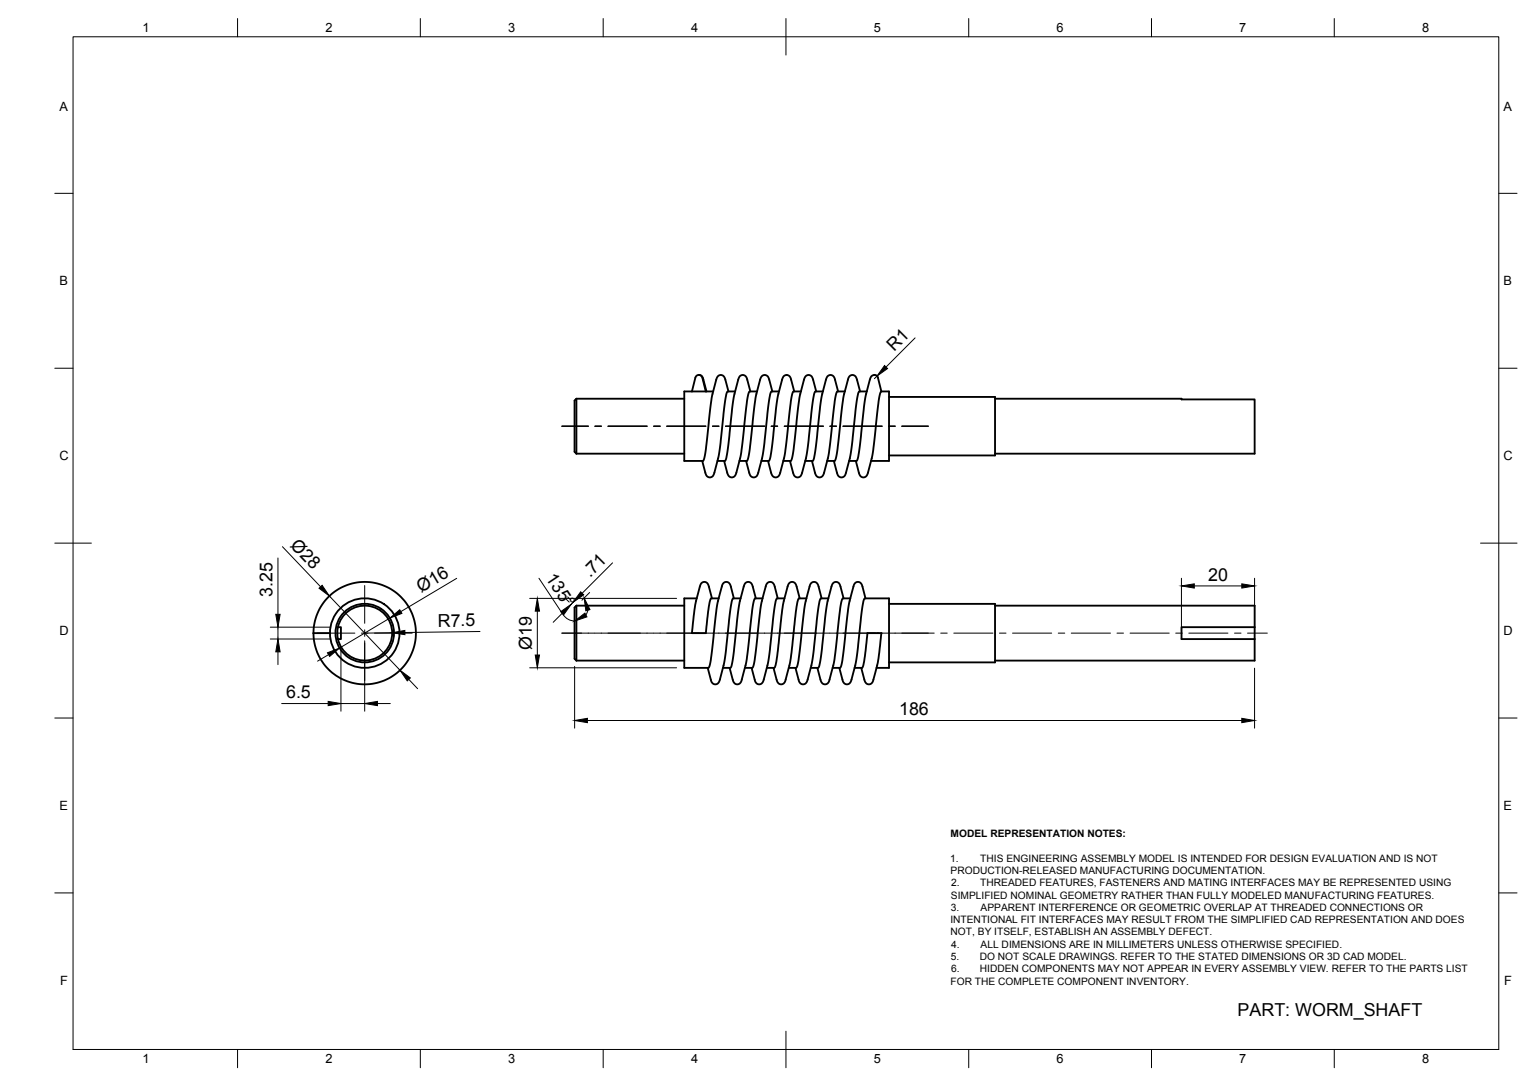
ISO-10303-21;
HEADER;
/* Generated by software containing ST-Developer
 * from STEP Tools, Inc. (www.steptools.com) 
 */

FILE_DESCRIPTION(
/* description */ ('STEP AP214'),
/* implementation_level */ '2;1');

FILE_NAME(
/* name */ 'Worm_Shaft.step',
/* time_stamp */ '2026-10-05T13:15:56-07:00',
/* author */ (''),
/* organization */ (''),
/* preprocessor_version */ 'ST-DEVELOPER v20.2',
/* originating_system */ 'Autodesk Translation Framework v15.15.0.0',
/* authorisation */ '');

FILE_SCHEMA (('AUTOMOTIVE_DESIGN { 1 0 10303 214 3 1 1 }'));
ENDSEC;

DATA;
#10=MECHANICAL_DESIGN_GEOMETRIC_PRESENTATION_REPRESENTATION('',(#1346),#37881);
#228=(
BOUNDED_CURVE()
B_SPLINE_CURVE(2,(#15162,#15163,#15164,#15165,#15166,#15167,#15168,#15169,
#15170,#15171,#15172,#15173,#15174,#15175,#15176,#15177,#15178,#15179,#15180,
#15181,#15182,#15183,#15184,#15185,#15186,#15187,#15188,#15189,#15190,#15191,
#15192,#15193,#15194,#15195,#15196,#15197,#15198,#15199,#15200,#15201,#15202,
#15203,#15204,#15205,#15206,#15207,#15208,#15209,#15210,#15211,#15212,#15213,
#15214,#15215,#15216,#15217,#15218,#15219,#15220,#15221,#15222,#15223,#15224,
#15225,#15226,#15227,#15228,#15229,#15230,#15231,#15232,#15233,#15234,#15235,
#15236,#15237,#15238,#15239,#15240,#15241,#15242,#15243,#15244,#15245,#15246,
#15247,#15248,#15249,#15250,#15251,#15252,#15253,#15254,#15255,#15256,#15257,
#15258,#15259,#15260,#15261,#15262,#15263,#15264,#15265,#15266,#15267,#15268,
#15269,#15270,#15271,#15272,#15273,#15274),.UNSPECIFIED.,.F.,.F.)
B_SPLINE_CURVE_WITH_KNOTS((3,2,2,2,2,2,2,2,2,2,2,2,2,2,2,2,2,2,2,2,2,2,
2,2,2,2,2,2,2,2,2,2,2,2,2,2,2,2,2,2,2,2,2,2,2,2,2,2,2,2,2,2,2,2,2,2,3),
(0.,0.0178571428571429,0.0357142857142857,0.0535714285714286,0.0714285714285714,
0.0892857142857143,0.107142857142857,0.125,0.142857142857143,0.160714285714286,
0.178571428571429,0.196428571428571,0.214285714285714,0.232142857142857,
0.25,0.267857142857143,0.285714285714286,0.303571428571429,0.321428571428571,
0.339285714285714,0.357142857142857,0.375,0.392857142857143,0.410714285714286,
0.428571428571429,0.446428571428571,0.464285714285714,0.482142857142857,
0.5,0.517857142857143,0.535714285714286,0.553571428571429,0.571428571428571,
0.589285714285714,0.607142857142857,0.625,0.642857142857143,0.660714285714286,
0.678571428571429,0.696428571428571,0.714285714285714,0.732142857142857,
0.75,0.767857142857143,0.785714285714286,0.803571428571429,0.821428571428571,
0.839285714285714,0.857142857142857,0.875,0.892857142857143,0.910714285714286,
0.928571428571429,0.946428571428571,0.964285714285714,0.982142857142857,
1.),.UNSPECIFIED.)
CURVE()
GEOMETRIC_REPRESENTATION_ITEM()
RATIONAL_B_SPLINE_CURVE((1.,0.974927912181824,1.,0.974927912181824,1.,0.974927912181824,
1.,0.974927912181824,1.,0.974927912181824,1.,0.974927912181824,1.,0.974927912181824,
1.,0.974927912181824,1.,0.974927912181824,1.,0.974927912181824,1.,0.974927912181824,
1.,0.974927912181824,1.,0.974927912181824,1.,0.974927912181824,1.,0.974927912181824,
1.,0.974927912181824,1.,0.974927912181824,1.,0.974927912181824,1.,0.974927912181824,
1.,0.974927912181824,1.,0.974927912181824,1.,0.974927912181824,1.,0.974927912181824,
1.,0.974927912181824,1.,0.974927912181824,1.,0.974927912181824,1.,0.974927912181824,
1.,0.974927912181824,1.,0.974927912181824,1.,0.974927912181824,1.,0.974927912181824,
1.,0.974927912181824,1.,0.974927912181824,1.,0.974927912181824,1.,0.974927912181824,
1.,0.974927912181824,1.,0.974927912181824,1.,0.974927912181824,1.,0.974927912181824,
1.,0.974927912181824,1.,0.974927912181824,1.,0.974927912181824,1.,0.974927912181824,
1.,0.974927912181824,1.,0.974927912181824,1.,0.974927912181824,1.,0.974927912181824,
1.,0.974927912181824,1.,0.974927912181824,1.,0.974927912181824,1.,0.974927912181824,
1.,0.974927912181824,1.,0.974927912181824,1.,0.974927912181824,1.,0.974927912181824,
1.,0.974927912181824,1.))
REPRESENTATION_ITEM('')
);
#229=(
BOUNDED_CURVE()
B_SPLINE_CURVE(2,(#15729,#15730,#15731,#15732,#15733,#15734,#15735,#15736,
#15737,#15738,#15739,#15740,#15741,#15742,#15743,#15744,#15745,#15746,#15747,
#15748,#15749,#15750,#15751,#15752,#15753,#15754,#15755,#15756,#15757,#15758,
#15759,#15760,#15761,#15762,#15763,#15764,#15765,#15766,#15767,#15768,#15769,
#15770,#15771,#15772,#15773,#15774,#15775,#15776,#15777,#15778,#15779,#15780,
#15781,#15782,#15783,#15784,#15785,#15786,#15787,#15788,#15789,#15790,#15791,
#15792,#15793,#15794,#15795,#15796,#15797,#15798,#15799,#15800,#15801,#15802,
#15803,#15804,#15805,#15806,#15807,#15808,#15809,#15810,#15811,#15812,#15813,
#15814,#15815,#15816,#15817,#15818,#15819,#15820,#15821,#15822,#15823,#15824,
#15825,#15826,#15827,#15828,#15829,#15830,#15831,#15832,#15833,#15834,#15835,
#15836,#15837,#15838,#15839,#15840,#15841),.UNSPECIFIED.,.F.,.F.)
B_SPLINE_CURVE_WITH_KNOTS((3,2,2,2,2,2,2,2,2,2,2,2,2,2,2,2,2,2,2,2,2,2,
2,2,2,2,2,2,2,2,2,2,2,2,2,2,2,2,2,2,2,2,2,2,2,2,2,2,2,2,2,2,2,2,2,2,3),
(0.,0.0178571428571429,0.0357142857142857,0.0535714285714286,0.0714285714285714,
0.0892857142857143,0.107142857142857,0.125,0.142857142857143,0.160714285714286,
0.178571428571429,0.196428571428571,0.214285714285714,0.232142857142857,
0.25,0.267857142857143,0.285714285714286,0.303571428571429,0.321428571428571,
0.339285714285714,0.357142857142857,0.375,0.392857142857143,0.410714285714286,
0.428571428571429,0.446428571428571,0.464285714285714,0.482142857142857,
0.5,0.517857142857143,0.535714285714286,0.553571428571429,0.571428571428571,
0.589285714285714,0.607142857142857,0.625,0.642857142857143,0.660714285714286,
0.678571428571429,0.696428571428571,0.714285714285714,0.732142857142857,
0.75,0.767857142857143,0.785714285714286,0.803571428571429,0.821428571428571,
0.839285714285714,0.857142857142857,0.875,0.892857142857143,0.910714285714286,
0.928571428571429,0.946428571428571,0.964285714285714,0.982142857142857,
1.),.UNSPECIFIED.)
CURVE()
GEOMETRIC_REPRESENTATION_ITEM()
RATIONAL_B_SPLINE_CURVE((1.,0.974927912181824,1.,0.974927912181824,1.,0.974927912181824,
1.,0.974927912181824,1.,0.974927912181824,1.,0.974927912181824,1.,0.974927912181824,
1.,0.974927912181824,1.,0.974927912181824,1.,0.974927912181824,1.,0.974927912181824,
1.,0.974927912181824,1.,0.974927912181824,1.,0.974927912181824,1.,0.974927912181824,
1.,0.974927912181824,1.,0.974927912181824,1.,0.974927912181824,1.,0.974927912181824,
1.,0.974927912181824,1.,0.974927912181824,1.,0.974927912181824,1.,0.974927912181824,
1.,0.974927912181824,1.,0.974927912181824,1.,0.974927912181824,1.,0.974927912181824,
1.,0.974927912181824,1.,0.974927912181824,1.,0.974927912181824,1.,0.974927912181824,
1.,0.974927912181824,1.,0.974927912181824,1.,0.974927912181824,1.,0.974927912181824,
1.,0.974927912181824,1.,0.974927912181824,1.,0.974927912181824,1.,0.974927912181824,
1.,0.974927912181824,1.,0.974927912181824,1.,0.974927912181824,1.,0.974927912181824,
1.,0.974927912181824,1.,0.974927912181824,1.,0.974927912181824,1.,0.974927912181824,
1.,0.974927912181824,1.,0.974927912181824,1.,0.974927912181824,1.,0.974927912181824,
1.,0.974927912181824,1.,0.974927912181824,1.,0.974927912181824,1.,0.974927912181824,
1.,0.974927912181824,1.))
REPRESENTATION_ITEM('')
);
#230=(
BOUNDED_CURVE()
B_SPLINE_CURVE(2,(#16301,#16302,#16303,#16304,#16305,#16306,#16307,#16308,
#16309,#16310,#16311,#16312,#16313,#16314,#16315,#16316,#16317,#16318,#16319,
#16320,#16321,#16322,#16323,#16324,#16325,#16326,#16327,#16328,#16329,#16330,
#16331,#16332,#16333,#16334,#16335,#16336,#16337,#16338,#16339,#16340,#16341,
#16342,#16343,#16344,#16345,#16346,#16347,#16348,#16349,#16350,#16351,#16352,
#16353,#16354,#16355,#16356,#16357,#16358,#16359,#16360,#16361,#16362,#16363,
#16364,#16365,#16366,#16367,#16368,#16369,#16370,#16371,#16372,#16373,#16374,
#16375,#16376,#16377,#16378,#16379,#16380,#16381,#16382,#16383,#16384,#16385,
#16386,#16387,#16388,#16389,#16390,#16391,#16392,#16393,#16394,#16395,#16396,
#16397,#16398,#16399,#16400,#16401,#16402,#16403,#16404,#16405,#16406,#16407,
#16408,#16409,#16410,#16411,#16412,#16413),.UNSPECIFIED.,.F.,.F.)
B_SPLINE_CURVE_WITH_KNOTS((3,2,2,2,2,2,2,2,2,2,2,2,2,2,2,2,2,2,2,2,2,2,
2,2,2,2,2,2,2,2,2,2,2,2,2,2,2,2,2,2,2,2,2,2,2,2,2,2,2,2,2,2,2,2,2,2,3),
(0.,0.0178571428571429,0.0357142857142857,0.0535714285714286,0.0714285714285714,
0.0892857142857143,0.107142857142857,0.125,0.142857142857143,0.160714285714286,
0.178571428571429,0.196428571428571,0.214285714285714,0.232142857142857,
0.25,0.267857142857143,0.285714285714286,0.303571428571429,0.321428571428571,
0.339285714285714,0.357142857142857,0.375,0.392857142857143,0.410714285714286,
0.428571428571429,0.446428571428571,0.464285714285714,0.482142857142857,
0.5,0.517857142857143,0.535714285714286,0.553571428571429,0.571428571428571,
0.589285714285714,0.607142857142857,0.625,0.642857142857143,0.660714285714286,
0.678571428571429,0.696428571428571,0.714285714285714,0.732142857142857,
0.75,0.767857142857143,0.785714285714286,0.803571428571429,0.821428571428571,
0.839285714285714,0.857142857142857,0.875,0.892857142857143,0.910714285714286,
0.928571428571429,0.946428571428571,0.964285714285714,0.982142857142857,
1.),.UNSPECIFIED.)
CURVE()
GEOMETRIC_REPRESENTATION_ITEM()
RATIONAL_B_SPLINE_CURVE((1.,0.974927912181824,1.,0.974927912181824,1.,0.974927912181824,
1.,0.974927912181824,1.,0.974927912181824,1.,0.974927912181824,1.,0.974927912181824,
1.,0.974927912181824,1.,0.974927912181824,1.,0.974927912181824,1.,0.974927912181824,
1.,0.974927912181824,1.,0.974927912181824,1.,0.974927912181824,1.,0.974927912181824,
1.,0.974927912181824,1.,0.974927912181824,1.,0.974927912181824,1.,0.974927912181824,
1.,0.974927912181824,1.,0.974927912181824,1.,0.974927912181824,1.,0.974927912181824,
1.,0.974927912181824,1.,0.974927912181824,1.,0.974927912181824,1.,0.974927912181824,
1.,0.974927912181824,1.,0.974927912181824,1.,0.974927912181824,1.,0.974927912181824,
1.,0.974927912181824,1.,0.974927912181824,1.,0.974927912181824,1.,0.974927912181824,
1.,0.974927912181824,1.,0.974927912181824,1.,0.974927912181824,1.,0.974927912181824,
1.,0.974927912181824,1.,0.974927912181824,1.,0.974927912181824,1.,0.974927912181824,
1.,0.974927912181824,1.,0.974927912181824,1.,0.974927912181824,1.,0.974927912181824,
1.,0.974927912181824,1.,0.974927912181824,1.,0.974927912181824,1.,0.974927912181824,
1.,0.974927912181824,1.,0.974927912181824,1.,0.974927912181824,1.,0.974927912181824,
1.,0.974927912181824,1.))
REPRESENTATION_ITEM('')
);
#231=(
BOUNDED_CURVE()
B_SPLINE_CURVE(2,(#16866,#16867,#16868,#16869,#16870,#16871,#16872,#16873,
#16874,#16875,#16876,#16877,#16878,#16879,#16880,#16881,#16882,#16883,#16884,
#16885,#16886,#16887,#16888,#16889,#16890,#16891,#16892,#16893,#16894,#16895,
#16896,#16897,#16898,#16899,#16900,#16901,#16902,#16903,#16904,#16905,#16906,
#16907,#16908,#16909,#16910,#16911,#16912,#16913,#16914,#16915,#16916,#16917,
#16918,#16919,#16920,#16921,#16922,#16923,#16924,#16925,#16926,#16927,#16928,
#16929,#16930,#16931,#16932,#16933,#16934,#16935,#16936,#16937,#16938,#16939,
#16940,#16941,#16942,#16943,#16944,#16945,#16946,#16947,#16948,#16949,#16950,
#16951,#16952,#16953,#16954,#16955,#16956,#16957,#16958,#16959,#16960,#16961,
#16962,#16963,#16964,#16965,#16966,#16967,#16968,#16969,#16970,#16971,#16972,
#16973,#16974,#16975,#16976,#16977,#16978),.UNSPECIFIED.,.F.,.F.)
B_SPLINE_CURVE_WITH_KNOTS((3,2,2,2,2,2,2,2,2,2,2,2,2,2,2,2,2,2,2,2,2,2,
2,2,2,2,2,2,2,2,2,2,2,2,2,2,2,2,2,2,2,2,2,2,2,2,2,2,2,2,2,2,2,2,2,2,3),
(0.,0.0178571428571429,0.0357142857142857,0.0535714285714286,0.0714285714285714,
0.0892857142857143,0.107142857142857,0.125,0.142857142857143,0.160714285714286,
0.178571428571429,0.196428571428571,0.214285714285714,0.232142857142857,
0.25,0.267857142857143,0.285714285714286,0.303571428571429,0.321428571428571,
0.339285714285714,0.357142857142857,0.375,0.392857142857143,0.410714285714286,
0.428571428571429,0.446428571428571,0.464285714285714,0.482142857142857,
0.5,0.517857142857143,0.535714285714286,0.553571428571429,0.571428571428571,
0.589285714285714,0.607142857142857,0.625,0.642857142857143,0.660714285714286,
0.678571428571429,0.696428571428571,0.714285714285714,0.732142857142857,
0.75,0.767857142857143,0.785714285714286,0.803571428571429,0.821428571428571,
0.839285714285714,0.857142857142857,0.875,0.892857142857143,0.910714285714286,
0.928571428571429,0.946428571428571,0.964285714285714,0.982142857142857,
1.),.UNSPECIFIED.)
CURVE()
GEOMETRIC_REPRESENTATION_ITEM()
RATIONAL_B_SPLINE_CURVE((1.,0.974927912181824,1.,0.974927912181824,1.,0.974927912181824,
1.,0.974927912181824,1.,0.974927912181824,1.,0.974927912181824,1.,0.974927912181824,
1.,0.974927912181824,1.,0.974927912181824,1.,0.974927912181824,1.,0.974927912181824,
1.,0.974927912181824,1.,0.974927912181824,1.,0.974927912181824,1.,0.974927912181824,
1.,0.974927912181824,1.,0.974927912181824,1.,0.974927912181824,1.,0.974927912181824,
1.,0.974927912181824,1.,0.974927912181824,1.,0.974927912181824,1.,0.974927912181824,
1.,0.974927912181824,1.,0.974927912181824,1.,0.974927912181824,1.,0.974927912181824,
1.,0.974927912181824,1.,0.974927912181824,1.,0.974927912181824,1.,0.974927912181824,
1.,0.974927912181824,1.,0.974927912181824,1.,0.974927912181824,1.,0.974927912181824,
1.,0.974927912181824,1.,0.974927912181824,1.,0.974927912181824,1.,0.974927912181824,
1.,0.974927912181824,1.,0.974927912181824,1.,0.974927912181824,1.,0.974927912181824,
1.,0.974927912181824,1.,0.974927912181824,1.,0.974927912181824,1.,0.974927912181824,
1.,0.974927912181824,1.,0.974927912181824,1.,0.974927912181824,1.,0.974927912181824,
1.,0.974927912181824,1.,0.974927912181824,1.,0.974927912181824,1.,0.974927912181824,
1.,0.974927912181824,1.))
REPRESENTATION_ITEM('')
);
#322=(
BOUNDED_SURFACE()
B_SPLINE_SURFACE(1,2,((#14934,#14935,#14936,#14937,#14938,#14939,#14940,
#14941,#14942,#14943,#14944,#14945,#14946,#14947,#14948,#14949,#14950,#14951,
#14952,#14953,#14954,#14955,#14956,#14957,#14958,#14959,#14960,#14961,#14962,
#14963,#14964,#14965,#14966,#14967,#14968,#14969,#14970,#14971,#14972,#14973,
#14974,#14975,#14976,#14977,#14978,#14979,#14980,#14981,#14982,#14983,#14984,
#14985,#14986,#14987,#14988,#14989,#14990,#14991,#14992,#14993,#14994,#14995,
#14996,#14997,#14998,#14999,#15000,#15001,#15002,#15003,#15004,#15005,#15006,
#15007,#15008,#15009,#15010,#15011,#15012,#15013,#15014,#15015,#15016,#15017,
#15018,#15019,#15020,#15021,#15022,#15023,#15024,#15025,#15026,#15027,#15028,
#15029,#15030,#15031,#15032,#15033,#15034,#15035,#15036,#15037,#15038,#15039,
#15040,#15041,#15042,#15043,#15044,#15045,#15046),(#15047,#15048,#15049,
#15050,#15051,#15052,#15053,#15054,#15055,#15056,#15057,#15058,#15059,#15060,
#15061,#15062,#15063,#15064,#15065,#15066,#15067,#15068,#15069,#15070,#15071,
#15072,#15073,#15074,#15075,#15076,#15077,#15078,#15079,#15080,#15081,#15082,
#15083,#15084,#15085,#15086,#15087,#15088,#15089,#15090,#15091,#15092,#15093,
#15094,#15095,#15096,#15097,#15098,#15099,#15100,#15101,#15102,#15103,#15104,
#15105,#15106,#15107,#15108,#15109,#15110,#15111,#15112,#15113,#15114,#15115,
#15116,#15117,#15118,#15119,#15120,#15121,#15122,#15123,#15124,#15125,#15126,
#15127,#15128,#15129,#15130,#15131,#15132,#15133,#15134,#15135,#15136,#15137,
#15138,#15139,#15140,#15141,#15142,#15143,#15144,#15145,#15146,#15147,#15148,
#15149,#15150,#15151,#15152,#15153,#15154,#15155,#15156,#15157,#15158,#15159)),
 .UNSPECIFIED.,.F.,.F.,.F.)
B_SPLINE_SURFACE_WITH_KNOTS((2,2),(3,2,2,2,2,2,2,2,2,2,2,2,2,2,2,2,2,2,
2,2,2,2,2,2,2,2,2,2,2,2,2,2,2,2,2,2,2,2,2,2,2,2,2,2,2,2,2,2,2,2,2,2,2,2,
2,2,3),(0.,1.),(0.,0.0178571428571429,0.0357142857142857,0.0535714285714286,
0.0714285714285714,0.0892857142857143,0.107142857142857,0.125,0.142857142857143,
0.160714285714286,0.178571428571429,0.196428571428571,0.214285714285714,
0.232142857142857,0.25,0.267857142857143,0.285714285714286,0.303571428571429,
0.321428571428571,0.339285714285714,0.357142857142857,0.375,0.392857142857143,
0.410714285714286,0.428571428571429,0.446428571428571,0.464285714285714,
0.482142857142857,0.5,0.517857142857143,0.535714285714286,0.553571428571429,
0.571428571428571,0.589285714285714,0.607142857142857,0.625,0.642857142857143,
0.660714285714286,0.678571428571429,0.696428571428571,0.714285714285714,
0.732142857142857,0.75,0.767857142857143,0.785714285714286,0.803571428571429,
0.821428571428571,0.839285714285714,0.857142857142857,0.875,0.892857142857143,
0.910714285714286,0.928571428571429,0.946428571428571,0.964285714285714,
0.982142857142857,1.),.UNSPECIFIED.)
GEOMETRIC_REPRESENTATION_ITEM()
RATIONAL_B_SPLINE_SURFACE(((1.,0.974927912181824,1.,0.974927912181824,1.,
0.974927912181824,1.,0.974927912181824,1.,0.974927912181824,1.,0.974927912181824,
1.,0.974927912181824,1.,0.974927912181824,1.,0.974927912181824,1.,0.974927912181824,
1.,0.974927912181824,1.,0.974927912181824,1.,0.974927912181824,1.,0.974927912181824,
1.,0.974927912181824,1.,0.974927912181824,1.,0.974927912181824,1.,0.974927912181824,
1.,0.974927912181824,1.,0.974927912181824,1.,0.974927912181824,1.,0.974927912181824,
1.,0.974927912181824,1.,0.974927912181824,1.,0.974927912181824,1.,0.974927912181824,
1.,0.974927912181824,1.,0.974927912181824,1.,0.974927912181824,1.,0.974927912181824,
1.,0.974927912181824,1.,0.974927912181824,1.,0.974927912181824,1.,0.974927912181824,
1.,0.974927912181824,1.,0.974927912181824,1.,0.974927912181824,1.,0.974927912181824,
1.,0.974927912181824,1.,0.974927912181824,1.,0.974927912181824,1.,0.974927912181824,
1.,0.974927912181824,1.,0.974927912181824,1.,0.974927912181824,1.,0.974927912181824,
1.,0.974927912181824,1.,0.974927912181824,1.,0.974927912181824,1.,0.974927912181824,
1.,0.974927912181824,1.,0.974927912181824,1.,0.974927912181824,1.,0.974927912181824,
1.,0.974927912181824,1.,0.974927912181824,1.),(1.,0.974927912181824,1.,
0.974927912181824,1.,0.974927912181824,1.,0.974927912181824,1.,0.974927912181824,
1.,0.974927912181824,1.,0.974927912181824,1.,0.974927912181824,1.,0.974927912181824,
1.,0.974927912181824,1.,0.974927912181824,1.,0.974927912181824,1.,0.974927912181824,
1.,0.974927912181824,1.,0.974927912181824,1.,0.974927912181824,1.,0.974927912181824,
1.,0.974927912181824,1.,0.974927912181824,1.,0.974927912181824,1.,0.974927912181824,
1.,0.974927912181824,1.,0.974927912181824,1.,0.974927912181824,1.,0.974927912181824,
1.,0.974927912181824,1.,0.974927912181824,1.,0.974927912181824,1.,0.974927912181824,
1.,0.974927912181824,1.,0.974927912181824,1.,0.974927912181824,1.,0.974927912181824,
1.,0.974927912181824,1.,0.974927912181824,1.,0.974927912181824,1.,0.974927912181824,
1.,0.974927912181824,1.,0.974927912181824,1.,0.974927912181824,1.,0.974927912181824,
1.,0.974927912181824,1.,0.974927912181824,1.,0.974927912181824,1.,0.974927912181824,
1.,0.974927912181824,1.,0.974927912181824,1.,0.974927912181824,1.,0.974927912181824,
1.,0.974927912181824,1.,0.974927912181824,1.,0.974927912181824,1.,0.974927912181824,
1.,0.974927912181824,1.,0.974927912181824,1.,0.974927912181824,1.)))
REPRESENTATION_ITEM('')
SURFACE()
);
#323=(
BOUNDED_SURFACE()
B_SPLINE_SURFACE(3,2,((#15275,#15276,#15277,#15278,#15279,#15280,#15281,
#15282,#15283,#15284,#15285,#15286,#15287,#15288,#15289,#15290,#15291,#15292,
#15293,#15294,#15295,#15296,#15297,#15298,#15299,#15300,#15301,#15302,#15303,
#15304,#15305,#15306,#15307,#15308,#15309,#15310,#15311,#15312,#15313,#15314,
#15315,#15316,#15317,#15318,#15319,#15320,#15321,#15322,#15323,#15324,#15325,
#15326,#15327,#15328,#15329,#15330,#15331,#15332,#15333,#15334,#15335,#15336,
#15337,#15338,#15339,#15340,#15341,#15342,#15343,#15344,#15345,#15346,#15347,
#15348,#15349,#15350,#15351,#15352,#15353,#15354,#15355,#15356,#15357,#15358,
#15359,#15360,#15361,#15362,#15363,#15364,#15365,#15366,#15367,#15368,#15369,
#15370,#15371,#15372,#15373,#15374,#15375,#15376,#15377,#15378,#15379,#15380,
#15381,#15382,#15383,#15384,#15385,#15386,#15387),(#15388,#15389,#15390,
#15391,#15392,#15393,#15394,#15395,#15396,#15397,#15398,#15399,#15400,#15401,
#15402,#15403,#15404,#15405,#15406,#15407,#15408,#15409,#15410,#15411,#15412,
#15413,#15414,#15415,#15416,#15417,#15418,#15419,#15420,#15421,#15422,#15423,
#15424,#15425,#15426,#15427,#15428,#15429,#15430,#15431,#15432,#15433,#15434,
#15435,#15436,#15437,#15438,#15439,#15440,#15441,#15442,#15443,#15444,#15445,
#15446,#15447,#15448,#15449,#15450,#15451,#15452,#15453,#15454,#15455,#15456,
#15457,#15458,#15459,#15460,#15461,#15462,#15463,#15464,#15465,#15466,#15467,
#15468,#15469,#15470,#15471,#15472,#15473,#15474,#15475,#15476,#15477,#15478,
#15479,#15480,#15481,#15482,#15483,#15484,#15485,#15486,#15487,#15488,#15489,
#15490,#15491,#15492,#15493,#15494,#15495,#15496,#15497,#15498,#15499,#15500),
(#15501,#15502,#15503,#15504,#15505,#15506,#15507,#15508,#15509,#15510,
#15511,#15512,#15513,#15514,#15515,#15516,#15517,#15518,#15519,#15520,#15521,
#15522,#15523,#15524,#15525,#15526,#15527,#15528,#15529,#15530,#15531,#15532,
#15533,#15534,#15535,#15536,#15537,#15538,#15539,#15540,#15541,#15542,#15543,
#15544,#15545,#15546,#15547,#15548,#15549,#15550,#15551,#15552,#15553,#15554,
#15555,#15556,#15557,#15558,#15559,#15560,#15561,#15562,#15563,#15564,#15565,
#15566,#15567,#15568,#15569,#15570,#15571,#15572,#15573,#15574,#15575,#15576,
#15577,#15578,#15579,#15580,#15581,#15582,#15583,#15584,#15585,#15586,#15587,
#15588,#15589,#15590,#15591,#15592,#15593,#15594,#15595,#15596,#15597,#15598,
#15599,#15600,#15601,#15602,#15603,#15604,#15605,#15606,#15607,#15608,#15609,
#15610,#15611,#15612,#15613),(#15614,#15615,#15616,#15617,#15618,#15619,
#15620,#15621,#15622,#15623,#15624,#15625,#15626,#15627,#15628,#15629,#15630,
#15631,#15632,#15633,#15634,#15635,#15636,#15637,#15638,#15639,#15640,#15641,
#15642,#15643,#15644,#15645,#15646,#15647,#15648,#15649,#15650,#15651,#15652,
#15653,#15654,#15655,#15656,#15657,#15658,#15659,#15660,#15661,#15662,#15663,
#15664,#15665,#15666,#15667,#15668,#15669,#15670,#15671,#15672,#15673,#15674,
#15675,#15676,#15677,#15678,#15679,#15680,#15681,#15682,#15683,#15684,#15685,
#15686,#15687,#15688,#15689,#15690,#15691,#15692,#15693,#15694,#15695,#15696,
#15697,#15698,#15699,#15700,#15701,#15702,#15703,#15704,#15705,#15706,#15707,
#15708,#15709,#15710,#15711,#15712,#15713,#15714,#15715,#15716,#15717,#15718,
#15719,#15720,#15721,#15722,#15723,#15724,#15725,#15726)),.UNSPECIFIED.,
 .F.,.F.,.F.)
B_SPLINE_SURFACE_WITH_KNOTS((4,4),(3,2,2,2,2,2,2,2,2,2,2,2,2,2,2,2,2,2,
2,2,2,2,2,2,2,2,2,2,2,2,2,2,2,2,2,2,2,2,2,2,2,2,2,2,2,2,2,2,2,2,2,2,2,2,
2,2,3),(0.,1.),(0.,0.0178571428571429,0.0357142857142857,0.0535714285714286,
0.0714285714285714,0.0892857142857143,0.107142857142857,0.125,0.142857142857143,
0.160714285714286,0.178571428571429,0.196428571428571,0.214285714285714,
0.232142857142857,0.25,0.267857142857143,0.285714285714286,0.303571428571429,
0.321428571428571,0.339285714285714,0.357142857142857,0.375,0.392857142857143,
0.410714285714286,0.428571428571429,0.446428571428571,0.464285714285714,
0.482142857142857,0.5,0.517857142857143,0.535714285714286,0.553571428571429,
0.571428571428571,0.589285714285714,0.607142857142857,0.625,0.642857142857143,
0.660714285714286,0.678571428571429,0.696428571428571,0.714285714285714,
0.732142857142857,0.75,0.767857142857143,0.785714285714286,0.803571428571429,
0.821428571428571,0.839285714285714,0.857142857142857,0.875,0.892857142857143,
0.910714285714286,0.928571428571429,0.946428571428571,0.964285714285714,
0.982142857142857,1.),.UNSPECIFIED.)
GEOMETRIC_REPRESENTATION_ITEM()
RATIONAL_B_SPLINE_SURFACE(((1.,0.974927912181824,1.,0.974927912181824,1.,
0.974927912181824,1.,0.974927912181824,1.,0.974927912181824,1.,0.974927912181824,
1.,0.974927912181824,1.,0.974927912181824,1.,0.974927912181824,1.,0.974927912181824,
1.,0.974927912181824,1.,0.974927912181824,1.,0.974927912181824,1.,0.974927912181824,
1.,0.974927912181824,1.,0.974927912181824,1.,0.974927912181824,1.,0.974927912181824,
1.,0.974927912181824,1.,0.974927912181824,1.,0.974927912181824,1.,0.974927912181824,
1.,0.974927912181824,1.,0.974927912181824,1.,0.974927912181824,1.,0.974927912181824,
1.,0.974927912181824,1.,0.974927912181824,1.,0.974927912181824,1.,0.974927912181824,
1.,0.974927912181824,1.,0.974927912181824,1.,0.974927912181824,1.,0.974927912181824,
1.,0.974927912181824,1.,0.974927912181824,1.,0.974927912181824,1.,0.974927912181824,
1.,0.974927912181824,1.,0.974927912181824,1.,0.974927912181824,1.,0.974927912181824,
1.,0.974927912181824,1.,0.974927912181824,1.,0.974927912181824,1.,0.974927912181824,
1.,0.974927912181824,1.,0.974927912181824,1.,0.974927912181824,1.,0.974927912181824,
1.,0.974927912181824,1.,0.974927912181824,1.,0.974927912181824,1.,0.974927912181824,
1.,0.974927912181824,1.,0.974927912181824,1.),(0.49408353936993,0.481695833481332,
0.49408353936993,0.481695833481332,0.49408353936993,0.481695833481332,0.49408353936993,
0.481695833481332,0.49408353936993,0.481695833481332,0.49408353936993,0.481695833481332,
0.49408353936993,0.481695833481332,0.49408353936993,0.481695833481332,0.49408353936993,
0.481695833481332,0.49408353936993,0.481695833481332,0.49408353936993,0.481695833481332,
0.49408353936993,0.481695833481332,0.49408353936993,0.481695833481332,0.49408353936993,
0.481695833481332,0.49408353936993,0.481695833481332,0.49408353936993,0.481695833481332,
0.49408353936993,0.481695833481332,0.49408353936993,0.481695833481332,0.49408353936993,
0.481695833481332,0.49408353936993,0.481695833481332,0.49408353936993,0.481695833481332,
0.49408353936993,0.481695833481332,0.49408353936993,0.481695833481332,0.49408353936993,
0.481695833481332,0.49408353936993,0.481695833481332,0.49408353936993,0.481695833481332,
0.49408353936993,0.481695833481332,0.49408353936993,0.481695833481332,0.49408353936993,
0.481695833481332,0.49408353936993,0.481695833481332,0.49408353936993,0.481695833481332,
0.49408353936993,0.481695833481332,0.49408353936993,0.481695833481332,0.49408353936993,
0.481695833481332,0.49408353936993,0.481695833481332,0.49408353936993,0.481695833481332,
0.49408353936993,0.481695833481332,0.49408353936993,0.481695833481332,0.49408353936993,
0.481695833481332,0.49408353936993,0.481695833481332,0.49408353936993,0.481695833481332,
0.49408353936993,0.481695833481332,0.49408353936993,0.481695833481332,0.49408353936993,
0.481695833481332,0.49408353936993,0.481695833481332,0.49408353936993,0.481695833481332,
0.49408353936993,0.481695833481332,0.49408353936993,0.481695833481332,0.49408353936993,
0.481695833481332,0.49408353936993,0.481695833481332,0.49408353936993,0.481695833481332,
0.49408353936993,0.481695833481332,0.49408353936993,0.481695833481332,0.49408353936993,
0.481695833481332,0.49408353936993,0.481695833481332,0.49408353936993,0.481695833481332,
0.49408353936993),(0.49408353936993,0.481695833481332,0.49408353936993,
0.481695833481332,0.49408353936993,0.481695833481332,0.49408353936993,0.481695833481332,
0.49408353936993,0.481695833481332,0.49408353936993,0.481695833481332,0.49408353936993,
0.481695833481332,0.49408353936993,0.481695833481332,0.49408353936993,0.481695833481332,
0.49408353936993,0.481695833481332,0.49408353936993,0.481695833481332,0.49408353936993,
0.481695833481332,0.49408353936993,0.481695833481332,0.49408353936993,0.481695833481332,
0.49408353936993,0.481695833481332,0.49408353936993,0.481695833481332,0.49408353936993,
0.481695833481332,0.49408353936993,0.481695833481332,0.49408353936993,0.481695833481332,
0.49408353936993,0.481695833481332,0.49408353936993,0.481695833481332,0.49408353936993,
0.481695833481332,0.49408353936993,0.481695833481332,0.49408353936993,0.481695833481332,
0.49408353936993,0.481695833481332,0.49408353936993,0.481695833481332,0.49408353936993,
0.481695833481332,0.49408353936993,0.481695833481332,0.49408353936993,0.481695833481332,
0.49408353936993,0.481695833481332,0.49408353936993,0.481695833481332,0.49408353936993,
0.481695833481332,0.49408353936993,0.481695833481332,0.49408353936993,0.481695833481332,
0.49408353936993,0.481695833481332,0.49408353936993,0.481695833481332,0.49408353936993,
0.481695833481332,0.49408353936993,0.481695833481332,0.49408353936993,0.481695833481332,
0.49408353936993,0.481695833481332,0.49408353936993,0.481695833481332,0.49408353936993,
0.481695833481332,0.49408353936993,0.481695833481332,0.49408353936993,0.481695833481332,
0.49408353936993,0.481695833481332,0.49408353936993,0.481695833481332,0.49408353936993,
0.481695833481332,0.49408353936993,0.481695833481332,0.49408353936993,0.481695833481332,
0.49408353936993,0.481695833481332,0.49408353936993,0.481695833481332,0.49408353936993,
0.481695833481332,0.49408353936993,0.481695833481332,0.49408353936993,0.481695833481332,
0.49408353936993,0.481695833481332,0.49408353936993,0.481695833481332,0.49408353936993),
(1.,0.974927912181824,1.,0.974927912181824,1.,0.974927912181824,1.,0.974927912181824,
1.,0.974927912181824,1.,0.974927912181824,1.,0.974927912181824,1.,0.974927912181824,
1.,0.974927912181824,1.,0.974927912181824,1.,0.974927912181824,1.,0.974927912181824,
1.,0.974927912181824,1.,0.974927912181824,1.,0.974927912181824,1.,0.974927912181824,
1.,0.974927912181824,1.,0.974927912181824,1.,0.974927912181824,1.,0.974927912181824,
1.,0.974927912181824,1.,0.974927912181824,1.,0.974927912181824,1.,0.974927912181824,
1.,0.974927912181824,1.,0.974927912181824,1.,0.974927912181824,1.,0.974927912181824,
1.,0.974927912181824,1.,0.974927912181824,1.,0.974927912181824,1.,0.974927912181824,
1.,0.974927912181824,1.,0.974927912181824,1.,0.974927912181824,1.,0.974927912181824,
1.,0.974927912181824,1.,0.974927912181824,1.,0.974927912181824,1.,0.974927912181824,
1.,0.974927912181824,1.,0.974927912181824,1.,0.974927912181824,1.,0.974927912181824,
1.,0.974927912181824,1.,0.974927912181824,1.,0.974927912181824,1.,0.974927912181824,
1.,0.974927912181824,1.,0.974927912181824,1.,0.974927912181824,1.,0.974927912181824,
1.,0.974927912181824,1.,0.974927912181824,1.,0.974927912181824,1.,0.974927912181824,
1.)))
REPRESENTATION_ITEM('')
SURFACE()
);
#324=(
BOUNDED_SURFACE()
B_SPLINE_SURFACE(1,2,((#15842,#15843,#15844,#15845,#15846,#15847,#15848,
#15849,#15850,#15851,#15852,#15853,#15854,#15855,#15856,#15857,#15858,#15859,
#15860,#15861,#15862,#15863,#15864,#15865,#15866,#15867,#15868,#15869,#15870,
#15871,#15872,#15873,#15874,#15875,#15876,#15877,#15878,#15879,#15880,#15881,
#15882,#15883,#15884,#15885,#15886,#15887,#15888,#15889,#15890,#15891,#15892,
#15893,#15894,#15895,#15896,#15897,#15898,#15899,#15900,#15901,#15902,#15903,
#15904,#15905,#15906,#15907,#15908,#15909,#15910,#15911,#15912,#15913,#15914,
#15915,#15916,#15917,#15918,#15919,#15920,#15921,#15922,#15923,#15924,#15925,
#15926,#15927,#15928,#15929,#15930,#15931,#15932,#15933,#15934,#15935,#15936,
#15937,#15938,#15939,#15940,#15941,#15942,#15943,#15944,#15945,#15946,#15947,
#15948,#15949,#15950,#15951,#15952,#15953,#15954),(#15955,#15956,#15957,
#15958,#15959,#15960,#15961,#15962,#15963,#15964,#15965,#15966,#15967,#15968,
#15969,#15970,#15971,#15972,#15973,#15974,#15975,#15976,#15977,#15978,#15979,
#15980,#15981,#15982,#15983,#15984,#15985,#15986,#15987,#15988,#15989,#15990,
#15991,#15992,#15993,#15994,#15995,#15996,#15997,#15998,#15999,#16000,#16001,
#16002,#16003,#16004,#16005,#16006,#16007,#16008,#16009,#16010,#16011,#16012,
#16013,#16014,#16015,#16016,#16017,#16018,#16019,#16020,#16021,#16022,#16023,
#16024,#16025,#16026,#16027,#16028,#16029,#16030,#16031,#16032,#16033,#16034,
#16035,#16036,#16037,#16038,#16039,#16040,#16041,#16042,#16043,#16044,#16045,
#16046,#16047,#16048,#16049,#16050,#16051,#16052,#16053,#16054,#16055,#16056,
#16057,#16058,#16059,#16060,#16061,#16062,#16063,#16064,#16065,#16066,#16067)),
 .UNSPECIFIED.,.F.,.F.,.F.)
B_SPLINE_SURFACE_WITH_KNOTS((2,2),(3,2,2,2,2,2,2,2,2,2,2,2,2,2,2,2,2,2,
2,2,2,2,2,2,2,2,2,2,2,2,2,2,2,2,2,2,2,2,2,2,2,2,2,2,2,2,2,2,2,2,2,2,2,2,
2,2,3),(0.,1.),(0.,0.0178571428571429,0.0357142857142857,0.0535714285714286,
0.0714285714285714,0.0892857142857143,0.107142857142857,0.125,0.142857142857143,
0.160714285714286,0.178571428571429,0.196428571428571,0.214285714285714,
0.232142857142857,0.25,0.267857142857143,0.285714285714286,0.303571428571429,
0.321428571428571,0.339285714285714,0.357142857142857,0.375,0.392857142857143,
0.410714285714286,0.428571428571429,0.446428571428571,0.464285714285714,
0.482142857142857,0.5,0.517857142857143,0.535714285714286,0.553571428571429,
0.571428571428571,0.589285714285714,0.607142857142857,0.625,0.642857142857143,
0.660714285714286,0.678571428571429,0.696428571428571,0.714285714285714,
0.732142857142857,0.75,0.767857142857143,0.785714285714286,0.803571428571429,
0.821428571428571,0.839285714285714,0.857142857142857,0.875,0.892857142857143,
0.910714285714286,0.928571428571429,0.946428571428571,0.964285714285714,
0.982142857142857,1.),.UNSPECIFIED.)
GEOMETRIC_REPRESENTATION_ITEM()
RATIONAL_B_SPLINE_SURFACE(((1.,0.974927912181824,1.,0.974927912181824,1.,
0.974927912181824,1.,0.974927912181824,1.,0.974927912181824,1.,0.974927912181824,
1.,0.974927912181824,1.,0.974927912181824,1.,0.974927912181824,1.,0.974927912181824,
1.,0.974927912181824,1.,0.974927912181824,1.,0.974927912181824,1.,0.974927912181824,
1.,0.974927912181824,1.,0.974927912181824,1.,0.974927912181824,1.,0.974927912181824,
1.,0.974927912181824,1.,0.974927912181824,1.,0.974927912181824,1.,0.974927912181824,
1.,0.974927912181824,1.,0.974927912181824,1.,0.974927912181824,1.,0.974927912181824,
1.,0.974927912181824,1.,0.974927912181824,1.,0.974927912181824,1.,0.974927912181824,
1.,0.974927912181824,1.,0.974927912181824,1.,0.974927912181824,1.,0.974927912181824,
1.,0.974927912181824,1.,0.974927912181824,1.,0.974927912181824,1.,0.974927912181824,
1.,0.974927912181824,1.,0.974927912181824,1.,0.974927912181824,1.,0.974927912181824,
1.,0.974927912181824,1.,0.974927912181824,1.,0.974927912181824,1.,0.974927912181824,
1.,0.974927912181824,1.,0.974927912181824,1.,0.974927912181824,1.,0.974927912181824,
1.,0.974927912181824,1.,0.974927912181824,1.,0.974927912181824,1.,0.974927912181824,
1.,0.974927912181824,1.,0.974927912181824,1.),(1.,0.974927912181824,1.,
0.974927912181824,1.,0.974927912181824,1.,0.974927912181824,1.,0.974927912181824,
1.,0.974927912181824,1.,0.974927912181824,1.,0.974927912181824,1.,0.974927912181824,
1.,0.974927912181824,1.,0.974927912181824,1.,0.974927912181824,1.,0.974927912181824,
1.,0.974927912181824,1.,0.974927912181824,1.,0.974927912181824,1.,0.974927912181824,
1.,0.974927912181824,1.,0.974927912181824,1.,0.974927912181824,1.,0.974927912181824,
1.,0.974927912181824,1.,0.974927912181824,1.,0.974927912181824,1.,0.974927912181824,
1.,0.974927912181824,1.,0.974927912181824,1.,0.974927912181824,1.,0.974927912181824,
1.,0.974927912181824,1.,0.974927912181824,1.,0.974927912181824,1.,0.974927912181824,
1.,0.974927912181824,1.,0.974927912181824,1.,0.974927912181824,1.,0.974927912181824,
1.,0.974927912181824,1.,0.974927912181824,1.,0.974927912181824,1.,0.974927912181824,
1.,0.974927912181824,1.,0.974927912181824,1.,0.974927912181824,1.,0.974927912181824,
1.,0.974927912181824,1.,0.974927912181824,1.,0.974927912181824,1.,0.974927912181824,
1.,0.974927912181824,1.,0.974927912181824,1.,0.974927912181824,1.,0.974927912181824,
1.,0.974927912181824,1.,0.974927912181824,1.,0.974927912181824,1.)))
REPRESENTATION_ITEM('')
SURFACE()
);
#325=(
BOUNDED_SURFACE()
B_SPLINE_SURFACE(1,2,((#16075,#16076,#16077,#16078,#16079,#16080,#16081,
#16082,#16083,#16084,#16085,#16086,#16087,#16088,#16089,#16090,#16091,#16092,
#16093,#16094,#16095,#16096,#16097,#16098,#16099,#16100,#16101,#16102,#16103,
#16104,#16105,#16106,#16107,#16108,#16109,#16110,#16111,#16112,#16113,#16114,
#16115,#16116,#16117,#16118,#16119,#16120,#16121,#16122,#16123,#16124,#16125,
#16126,#16127,#16128,#16129,#16130,#16131,#16132,#16133,#16134,#16135,#16136,
#16137,#16138,#16139,#16140,#16141,#16142,#16143,#16144,#16145,#16146,#16147,
#16148,#16149,#16150,#16151,#16152,#16153,#16154,#16155,#16156,#16157,#16158,
#16159,#16160,#16161,#16162,#16163,#16164,#16165,#16166,#16167,#16168,#16169,
#16170,#16171,#16172,#16173,#16174,#16175,#16176,#16177,#16178,#16179,#16180,
#16181,#16182,#16183,#16184,#16185,#16186,#16187),(#16188,#16189,#16190,
#16191,#16192,#16193,#16194,#16195,#16196,#16197,#16198,#16199,#16200,#16201,
#16202,#16203,#16204,#16205,#16206,#16207,#16208,#16209,#16210,#16211,#16212,
#16213,#16214,#16215,#16216,#16217,#16218,#16219,#16220,#16221,#16222,#16223,
#16224,#16225,#16226,#16227,#16228,#16229,#16230,#16231,#16232,#16233,#16234,
#16235,#16236,#16237,#16238,#16239,#16240,#16241,#16242,#16243,#16244,#16245,
#16246,#16247,#16248,#16249,#16250,#16251,#16252,#16253,#16254,#16255,#16256,
#16257,#16258,#16259,#16260,#16261,#16262,#16263,#16264,#16265,#16266,#16267,
#16268,#16269,#16270,#16271,#16272,#16273,#16274,#16275,#16276,#16277,#16278,
#16279,#16280,#16281,#16282,#16283,#16284,#16285,#16286,#16287,#16288,#16289,
#16290,#16291,#16292,#16293,#16294,#16295,#16296,#16297,#16298,#16299,#16300)),
 .UNSPECIFIED.,.F.,.F.,.F.)
B_SPLINE_SURFACE_WITH_KNOTS((2,2),(3,2,2,2,2,2,2,2,2,2,2,2,2,2,2,2,2,2,
2,2,2,2,2,2,2,2,2,2,2,2,2,2,2,2,2,2,2,2,2,2,2,2,2,2,2,2,2,2,2,2,2,2,2,2,
2,2,3),(0.,1.),(0.,0.0178571428571429,0.0357142857142857,0.0535714285714286,
0.0714285714285714,0.0892857142857143,0.107142857142857,0.125,0.142857142857143,
0.160714285714286,0.178571428571429,0.196428571428571,0.214285714285714,
0.232142857142857,0.25,0.267857142857143,0.285714285714286,0.303571428571429,
0.321428571428571,0.339285714285714,0.357142857142857,0.375,0.392857142857143,
0.410714285714286,0.428571428571429,0.446428571428571,0.464285714285714,
0.482142857142857,0.5,0.517857142857143,0.535714285714286,0.553571428571429,
0.571428571428571,0.589285714285714,0.607142857142857,0.625,0.642857142857143,
0.660714285714286,0.678571428571429,0.696428571428571,0.714285714285714,
0.732142857142857,0.75,0.767857142857143,0.785714285714286,0.803571428571429,
0.821428571428571,0.839285714285714,0.857142857142857,0.875,0.892857142857143,
0.910714285714286,0.928571428571429,0.946428571428571,0.964285714285714,
0.982142857142857,1.),.UNSPECIFIED.)
GEOMETRIC_REPRESENTATION_ITEM()
RATIONAL_B_SPLINE_SURFACE(((1.,0.974927912181824,1.,0.974927912181824,1.,
0.974927912181824,1.,0.974927912181824,1.,0.974927912181824,1.,0.974927912181824,
1.,0.974927912181824,1.,0.974927912181824,1.,0.974927912181824,1.,0.974927912181824,
1.,0.974927912181824,1.,0.974927912181824,1.,0.974927912181824,1.,0.974927912181824,
1.,0.974927912181824,1.,0.974927912181824,1.,0.974927912181824,1.,0.974927912181824,
1.,0.974927912181824,1.,0.974927912181824,1.,0.974927912181824,1.,0.974927912181824,
1.,0.974927912181824,1.,0.974927912181824,1.,0.974927912181824,1.,0.974927912181824,
1.,0.974927912181824,1.,0.974927912181824,1.,0.974927912181824,1.,0.974927912181824,
1.,0.974927912181824,1.,0.974927912181824,1.,0.974927912181824,1.,0.974927912181824,
1.,0.974927912181824,1.,0.974927912181824,1.,0.974927912181824,1.,0.974927912181824,
1.,0.974927912181824,1.,0.974927912181824,1.,0.974927912181824,1.,0.974927912181824,
1.,0.974927912181824,1.,0.974927912181824,1.,0.974927912181824,1.,0.974927912181824,
1.,0.974927912181824,1.,0.974927912181824,1.,0.974927912181824,1.,0.974927912181824,
1.,0.974927912181824,1.,0.974927912181824,1.,0.974927912181824,1.,0.974927912181824,
1.,0.974927912181824,1.,0.974927912181824,1.),(1.,0.974927912181824,1.,
0.974927912181824,1.,0.974927912181824,1.,0.974927912181824,1.,0.974927912181824,
1.,0.974927912181824,1.,0.974927912181824,1.,0.974927912181824,1.,0.974927912181824,
1.,0.974927912181824,1.,0.974927912181824,1.,0.974927912181824,1.,0.974927912181824,
1.,0.974927912181824,1.,0.974927912181824,1.,0.974927912181824,1.,0.974927912181824,
1.,0.974927912181824,1.,0.974927912181824,1.,0.974927912181824,1.,0.974927912181824,
1.,0.974927912181824,1.,0.974927912181824,1.,0.974927912181824,1.,0.974927912181824,
1.,0.974927912181824,1.,0.974927912181824,1.,0.974927912181824,1.,0.974927912181824,
1.,0.974927912181824,1.,0.974927912181824,1.,0.974927912181824,1.,0.974927912181824,
1.,0.974927912181824,1.,0.974927912181824,1.,0.974927912181824,1.,0.974927912181824,
1.,0.974927912181824,1.,0.974927912181824,1.,0.974927912181824,1.,0.974927912181824,
1.,0.974927912181824,1.,0.974927912181824,1.,0.974927912181824,1.,0.974927912181824,
1.,0.974927912181824,1.,0.974927912181824,1.,0.974927912181824,1.,0.974927912181824,
1.,0.974927912181824,1.,0.974927912181824,1.,0.974927912181824,1.,0.974927912181824,
1.,0.974927912181824,1.,0.974927912181824,1.,0.974927912181824,1.)))
REPRESENTATION_ITEM('')
SURFACE()
);
#326=(
BOUNDED_SURFACE()
B_SPLINE_SURFACE(3,2,((#16414,#16415,#16416,#16417,#16418,#16419,#16420,
#16421,#16422,#16423,#16424,#16425,#16426,#16427,#16428,#16429,#16430,#16431,
#16432,#16433,#16434,#16435,#16436,#16437,#16438,#16439,#16440,#16441,#16442,
#16443,#16444,#16445,#16446,#16447,#16448,#16449,#16450,#16451,#16452,#16453,
#16454,#16455,#16456,#16457,#16458,#16459,#16460,#16461,#16462,#16463,#16464,
#16465,#16466,#16467,#16468,#16469,#16470,#16471,#16472,#16473,#16474,#16475,
#16476,#16477,#16478,#16479,#16480,#16481,#16482,#16483,#16484,#16485,#16486,
#16487,#16488,#16489,#16490,#16491,#16492,#16493,#16494,#16495,#16496,#16497,
#16498,#16499,#16500,#16501,#16502,#16503,#16504,#16505,#16506,#16507,#16508,
#16509,#16510,#16511,#16512,#16513,#16514,#16515,#16516,#16517,#16518,#16519,
#16520,#16521,#16522,#16523,#16524,#16525,#16526),(#16527,#16528,#16529,
#16530,#16531,#16532,#16533,#16534,#16535,#16536,#16537,#16538,#16539,#16540,
#16541,#16542,#16543,#16544,#16545,#16546,#16547,#16548,#16549,#16550,#16551,
#16552,#16553,#16554,#16555,#16556,#16557,#16558,#16559,#16560,#16561,#16562,
#16563,#16564,#16565,#16566,#16567,#16568,#16569,#16570,#16571,#16572,#16573,
#16574,#16575,#16576,#16577,#16578,#16579,#16580,#16581,#16582,#16583,#16584,
#16585,#16586,#16587,#16588,#16589,#16590,#16591,#16592,#16593,#16594,#16595,
#16596,#16597,#16598,#16599,#16600,#16601,#16602,#16603,#16604,#16605,#16606,
#16607,#16608,#16609,#16610,#16611,#16612,#16613,#16614,#16615,#16616,#16617,
#16618,#16619,#16620,#16621,#16622,#16623,#16624,#16625,#16626,#16627,#16628,
#16629,#16630,#16631,#16632,#16633,#16634,#16635,#16636,#16637,#16638,#16639),
(#16640,#16641,#16642,#16643,#16644,#16645,#16646,#16647,#16648,#16649,
#16650,#16651,#16652,#16653,#16654,#16655,#16656,#16657,#16658,#16659,#16660,
#16661,#16662,#16663,#16664,#16665,#16666,#16667,#16668,#16669,#16670,#16671,
#16672,#16673,#16674,#16675,#16676,#16677,#16678,#16679,#16680,#16681,#16682,
#16683,#16684,#16685,#16686,#16687,#16688,#16689,#16690,#16691,#16692,#16693,
#16694,#16695,#16696,#16697,#16698,#16699,#16700,#16701,#16702,#16703,#16704,
#16705,#16706,#16707,#16708,#16709,#16710,#16711,#16712,#16713,#16714,#16715,
#16716,#16717,#16718,#16719,#16720,#16721,#16722,#16723,#16724,#16725,#16726,
#16727,#16728,#16729,#16730,#16731,#16732,#16733,#16734,#16735,#16736,#16737,
#16738,#16739,#16740,#16741,#16742,#16743,#16744,#16745,#16746,#16747,#16748,
#16749,#16750,#16751,#16752),(#16753,#16754,#16755,#16756,#16757,#16758,
#16759,#16760,#16761,#16762,#16763,#16764,#16765,#16766,#16767,#16768,#16769,
#16770,#16771,#16772,#16773,#16774,#16775,#16776,#16777,#16778,#16779,#16780,
#16781,#16782,#16783,#16784,#16785,#16786,#16787,#16788,#16789,#16790,#16791,
#16792,#16793,#16794,#16795,#16796,#16797,#16798,#16799,#16800,#16801,#16802,
#16803,#16804,#16805,#16806,#16807,#16808,#16809,#16810,#16811,#16812,#16813,
#16814,#16815,#16816,#16817,#16818,#16819,#16820,#16821,#16822,#16823,#16824,
#16825,#16826,#16827,#16828,#16829,#16830,#16831,#16832,#16833,#16834,#16835,
#16836,#16837,#16838,#16839,#16840,#16841,#16842,#16843,#16844,#16845,#16846,
#16847,#16848,#16849,#16850,#16851,#16852,#16853,#16854,#16855,#16856,#16857,
#16858,#16859,#16860,#16861,#16862,#16863,#16864,#16865)),.UNSPECIFIED.,
 .F.,.F.,.F.)
B_SPLINE_SURFACE_WITH_KNOTS((4,4),(3,2,2,2,2,2,2,2,2,2,2,2,2,2,2,2,2,2,
2,2,2,2,2,2,2,2,2,2,2,2,2,2,2,2,2,2,2,2,2,2,2,2,2,2,2,2,2,2,2,2,2,2,2,2,
2,2,3),(0.,1.),(0.,0.0178571428571429,0.0357142857142857,0.0535714285714286,
0.0714285714285714,0.0892857142857143,0.107142857142857,0.125,0.142857142857143,
0.160714285714286,0.178571428571429,0.196428571428571,0.214285714285714,
0.232142857142857,0.25,0.267857142857143,0.285714285714286,0.303571428571429,
0.321428571428571,0.339285714285714,0.357142857142857,0.375,0.392857142857143,
0.410714285714286,0.428571428571429,0.446428571428571,0.464285714285714,
0.482142857142857,0.5,0.517857142857143,0.535714285714286,0.553571428571429,
0.571428571428571,0.589285714285714,0.607142857142857,0.625,0.642857142857143,
0.660714285714286,0.678571428571429,0.696428571428571,0.714285714285714,
0.732142857142857,0.75,0.767857142857143,0.785714285714286,0.803571428571429,
0.821428571428571,0.839285714285714,0.857142857142857,0.875,0.892857142857143,
0.910714285714286,0.928571428571429,0.946428571428571,0.964285714285714,
0.982142857142857,1.),.UNSPECIFIED.)
GEOMETRIC_REPRESENTATION_ITEM()
RATIONAL_B_SPLINE_SURFACE(((1.,0.974927912181824,1.,0.974927912181824,1.,
0.974927912181824,1.,0.974927912181824,1.,0.974927912181824,1.,0.974927912181824,
1.,0.974927912181824,1.,0.974927912181824,1.,0.974927912181824,1.,0.974927912181824,
1.,0.974927912181824,1.,0.974927912181824,1.,0.974927912181824,1.,0.974927912181824,
1.,0.974927912181824,1.,0.974927912181824,1.,0.974927912181824,1.,0.974927912181824,
1.,0.974927912181824,1.,0.974927912181824,1.,0.974927912181824,1.,0.974927912181824,
1.,0.974927912181824,1.,0.974927912181824,1.,0.974927912181824,1.,0.974927912181824,
1.,0.974927912181824,1.,0.974927912181824,1.,0.974927912181824,1.,0.974927912181824,
1.,0.974927912181824,1.,0.974927912181824,1.,0.974927912181824,1.,0.974927912181824,
1.,0.974927912181824,1.,0.974927912181824,1.,0.974927912181824,1.,0.974927912181824,
1.,0.974927912181824,1.,0.974927912181824,1.,0.974927912181824,1.,0.974927912181824,
1.,0.974927912181824,1.,0.974927912181824,1.,0.974927912181824,1.,0.974927912181824,
1.,0.974927912181824,1.,0.974927912181824,1.,0.974927912181824,1.,0.974927912181824,
1.,0.974927912181824,1.,0.974927912181824,1.,0.974927912181824,1.,0.974927912181824,
1.,0.974927912181824,1.,0.974927912181824,1.),(0.49408353936993,0.481695833481332,
0.49408353936993,0.481695833481332,0.49408353936993,0.481695833481332,0.49408353936993,
0.481695833481332,0.49408353936993,0.481695833481332,0.49408353936993,0.481695833481332,
0.49408353936993,0.481695833481332,0.49408353936993,0.481695833481332,0.49408353936993,
0.481695833481332,0.49408353936993,0.481695833481332,0.49408353936993,0.481695833481332,
0.49408353936993,0.481695833481332,0.49408353936993,0.481695833481332,0.49408353936993,
0.481695833481332,0.49408353936993,0.481695833481332,0.49408353936993,0.481695833481332,
0.49408353936993,0.481695833481332,0.49408353936993,0.481695833481332,0.49408353936993,
0.481695833481332,0.49408353936993,0.481695833481332,0.49408353936993,0.481695833481332,
0.49408353936993,0.481695833481332,0.49408353936993,0.481695833481332,0.49408353936993,
0.481695833481332,0.49408353936993,0.481695833481332,0.49408353936993,0.481695833481332,
0.49408353936993,0.481695833481332,0.49408353936993,0.481695833481332,0.49408353936993,
0.481695833481332,0.49408353936993,0.481695833481332,0.49408353936993,0.481695833481332,
0.49408353936993,0.481695833481332,0.49408353936993,0.481695833481332,0.49408353936993,
0.481695833481332,0.49408353936993,0.481695833481332,0.49408353936993,0.481695833481332,
0.49408353936993,0.481695833481332,0.49408353936993,0.481695833481332,0.49408353936993,
0.481695833481332,0.49408353936993,0.481695833481332,0.49408353936993,0.481695833481332,
0.49408353936993,0.481695833481332,0.49408353936993,0.481695833481332,0.49408353936993,
0.481695833481332,0.49408353936993,0.481695833481332,0.49408353936993,0.481695833481332,
0.49408353936993,0.481695833481332,0.49408353936993,0.481695833481332,0.49408353936993,
0.481695833481332,0.49408353936993,0.481695833481332,0.49408353936993,0.481695833481332,
0.49408353936993,0.481695833481332,0.49408353936993,0.481695833481332,0.49408353936993,
0.481695833481332,0.49408353936993,0.481695833481332,0.49408353936993,0.481695833481332,
0.49408353936993),(0.49408353936993,0.481695833481332,0.49408353936993,
0.481695833481332,0.49408353936993,0.481695833481332,0.49408353936993,0.481695833481332,
0.49408353936993,0.481695833481332,0.49408353936993,0.481695833481332,0.49408353936993,
0.481695833481332,0.49408353936993,0.481695833481332,0.49408353936993,0.481695833481332,
0.49408353936993,0.481695833481332,0.49408353936993,0.481695833481332,0.49408353936993,
0.481695833481332,0.49408353936993,0.481695833481332,0.49408353936993,0.481695833481332,
0.49408353936993,0.481695833481332,0.49408353936993,0.481695833481332,0.49408353936993,
0.481695833481332,0.49408353936993,0.481695833481332,0.49408353936993,0.481695833481332,
0.49408353936993,0.481695833481332,0.49408353936993,0.481695833481332,0.49408353936993,
0.481695833481332,0.49408353936993,0.481695833481332,0.49408353936993,0.481695833481332,
0.49408353936993,0.481695833481332,0.49408353936993,0.481695833481332,0.49408353936993,
0.481695833481332,0.49408353936993,0.481695833481332,0.49408353936993,0.481695833481332,
0.49408353936993,0.481695833481332,0.49408353936993,0.481695833481332,0.49408353936993,
0.481695833481332,0.49408353936993,0.481695833481332,0.49408353936993,0.481695833481332,
0.49408353936993,0.481695833481332,0.49408353936993,0.481695833481332,0.49408353936993,
0.481695833481332,0.49408353936993,0.481695833481332,0.49408353936993,0.481695833481332,
0.49408353936993,0.481695833481332,0.49408353936993,0.481695833481332,0.49408353936993,
0.481695833481332,0.49408353936993,0.481695833481332,0.49408353936993,0.481695833481332,
0.49408353936993,0.481695833481332,0.49408353936993,0.481695833481332,0.49408353936993,
0.481695833481332,0.49408353936993,0.481695833481332,0.49408353936993,0.481695833481332,
0.49408353936993,0.481695833481332,0.49408353936993,0.481695833481332,0.49408353936993,
0.481695833481332,0.49408353936993,0.481695833481332,0.49408353936993,0.481695833481332,
0.49408353936993,0.481695833481332,0.49408353936993,0.481695833481332,0.49408353936993),
(1.,0.974927912181824,1.,0.974927912181824,1.,0.974927912181824,1.,0.974927912181824,
1.,0.974927912181824,1.,0.974927912181824,1.,0.974927912181824,1.,0.974927912181824,
1.,0.974927912181824,1.,0.974927912181824,1.,0.974927912181824,1.,0.974927912181824,
1.,0.974927912181824,1.,0.974927912181824,1.,0.974927912181824,1.,0.974927912181824,
1.,0.974927912181824,1.,0.974927912181824,1.,0.974927912181824,1.,0.974927912181824,
1.,0.974927912181824,1.,0.974927912181824,1.,0.974927912181824,1.,0.974927912181824,
1.,0.974927912181824,1.,0.974927912181824,1.,0.974927912181824,1.,0.974927912181824,
1.,0.974927912181824,1.,0.974927912181824,1.,0.974927912181824,1.,0.974927912181824,
1.,0.974927912181824,1.,0.974927912181824,1.,0.974927912181824,1.,0.974927912181824,
1.,0.974927912181824,1.,0.974927912181824,1.,0.974927912181824,1.,0.974927912181824,
1.,0.974927912181824,1.,0.974927912181824,1.,0.974927912181824,1.,0.974927912181824,
1.,0.974927912181824,1.,0.974927912181824,1.,0.974927912181824,1.,0.974927912181824,
1.,0.974927912181824,1.,0.974927912181824,1.,0.974927912181824,1.,0.974927912181824,
1.,0.974927912181824,1.,0.974927912181824,1.,0.974927912181824,1.,0.974927912181824,
1.)))
REPRESENTATION_ITEM('')
SURFACE()
);
#327=(
BOUNDED_SURFACE()
B_SPLINE_SURFACE(1,2,((#16979,#16980,#16981,#16982,#16983,#16984,#16985,
#16986,#16987,#16988,#16989,#16990,#16991,#16992,#16993,#16994,#16995,#16996,
#16997,#16998,#16999,#17000,#17001,#17002,#17003,#17004,#17005,#17006,#17007,
#17008,#17009,#17010,#17011,#17012,#17013,#17014,#17015,#17016,#17017,#17018,
#17019,#17020,#17021,#17022,#17023,#17024,#17025,#17026,#17027,#17028,#17029,
#17030,#17031,#17032,#17033,#17034,#17035,#17036,#17037,#17038,#17039,#17040,
#17041,#17042,#17043,#17044,#17045,#17046,#17047,#17048,#17049,#17050,#17051,
#17052,#17053,#17054,#17055,#17056,#17057,#17058,#17059,#17060,#17061,#17062,
#17063,#17064,#17065,#17066,#17067,#17068,#17069,#17070,#17071,#17072,#17073,
#17074,#17075,#17076,#17077,#17078,#17079,#17080,#17081,#17082,#17083,#17084,
#17085,#17086,#17087,#17088,#17089,#17090,#17091),(#17092,#17093,#17094,
#17095,#17096,#17097,#17098,#17099,#17100,#17101,#17102,#17103,#17104,#17105,
#17106,#17107,#17108,#17109,#17110,#17111,#17112,#17113,#17114,#17115,#17116,
#17117,#17118,#17119,#17120,#17121,#17122,#17123,#17124,#17125,#17126,#17127,
#17128,#17129,#17130,#17131,#17132,#17133,#17134,#17135,#17136,#17137,#17138,
#17139,#17140,#17141,#17142,#17143,#17144,#17145,#17146,#17147,#17148,#17149,
#17150,#17151,#17152,#17153,#17154,#17155,#17156,#17157,#17158,#17159,#17160,
#17161,#17162,#17163,#17164,#17165,#17166,#17167,#17168,#17169,#17170,#17171,
#17172,#17173,#17174,#17175,#17176,#17177,#17178,#17179,#17180,#17181,#17182,
#17183,#17184,#17185,#17186,#17187,#17188,#17189,#17190,#17191,#17192,#17193,
#17194,#17195,#17196,#17197,#17198,#17199,#17200,#17201,#17202,#17203,#17204)),
 .UNSPECIFIED.,.F.,.F.,.F.)
B_SPLINE_SURFACE_WITH_KNOTS((2,2),(3,2,2,2,2,2,2,2,2,2,2,2,2,2,2,2,2,2,
2,2,2,2,2,2,2,2,2,2,2,2,2,2,2,2,2,2,2,2,2,2,2,2,2,2,2,2,2,2,2,2,2,2,2,2,
2,2,3),(0.,1.),(0.,0.0178571428571429,0.0357142857142857,0.0535714285714286,
0.0714285714285714,0.0892857142857143,0.107142857142857,0.125,0.142857142857143,
0.160714285714286,0.178571428571429,0.196428571428571,0.214285714285714,
0.232142857142857,0.25,0.267857142857143,0.285714285714286,0.303571428571429,
0.321428571428571,0.339285714285714,0.357142857142857,0.375,0.392857142857143,
0.410714285714286,0.428571428571429,0.446428571428571,0.464285714285714,
0.482142857142857,0.5,0.517857142857143,0.535714285714286,0.553571428571429,
0.571428571428571,0.589285714285714,0.607142857142857,0.625,0.642857142857143,
0.660714285714286,0.678571428571429,0.696428571428571,0.714285714285714,
0.732142857142857,0.75,0.767857142857143,0.785714285714286,0.803571428571429,
0.821428571428571,0.839285714285714,0.857142857142857,0.875,0.892857142857143,
0.910714285714286,0.928571428571429,0.946428571428571,0.964285714285714,
0.982142857142857,1.),.UNSPECIFIED.)
GEOMETRIC_REPRESENTATION_ITEM()
RATIONAL_B_SPLINE_SURFACE(((1.,0.974927912181824,1.,0.974927912181824,1.,
0.974927912181824,1.,0.974927912181824,1.,0.974927912181824,1.,0.974927912181824,
1.,0.974927912181824,1.,0.974927912181824,1.,0.974927912181824,1.,0.974927912181824,
1.,0.974927912181824,1.,0.974927912181824,1.,0.974927912181824,1.,0.974927912181824,
1.,0.974927912181824,1.,0.974927912181824,1.,0.974927912181824,1.,0.974927912181824,
1.,0.974927912181824,1.,0.974927912181824,1.,0.974927912181824,1.,0.974927912181824,
1.,0.974927912181824,1.,0.974927912181824,1.,0.974927912181824,1.,0.974927912181824,
1.,0.974927912181824,1.,0.974927912181824,1.,0.974927912181824,1.,0.974927912181824,
1.,0.974927912181824,1.,0.974927912181824,1.,0.974927912181824,1.,0.974927912181824,
1.,0.974927912181824,1.,0.974927912181824,1.,0.974927912181824,1.,0.974927912181824,
1.,0.974927912181824,1.,0.974927912181824,1.,0.974927912181824,1.,0.974927912181824,
1.,0.974927912181824,1.,0.974927912181824,1.,0.974927912181824,1.,0.974927912181824,
1.,0.974927912181824,1.,0.974927912181824,1.,0.974927912181824,1.,0.974927912181824,
1.,0.974927912181824,1.,0.974927912181824,1.,0.974927912181824,1.,0.974927912181824,
1.,0.974927912181824,1.,0.974927912181824,1.),(1.,0.974927912181824,1.,
0.974927912181824,1.,0.974927912181824,1.,0.974927912181824,1.,0.974927912181824,
1.,0.974927912181824,1.,0.974927912181824,1.,0.974927912181824,1.,0.974927912181824,
1.,0.974927912181824,1.,0.974927912181824,1.,0.974927912181824,1.,0.974927912181824,
1.,0.974927912181824,1.,0.974927912181824,1.,0.974927912181824,1.,0.974927912181824,
1.,0.974927912181824,1.,0.974927912181824,1.,0.974927912181824,1.,0.974927912181824,
1.,0.974927912181824,1.,0.974927912181824,1.,0.974927912181824,1.,0.974927912181824,
1.,0.974927912181824,1.,0.974927912181824,1.,0.974927912181824,1.,0.974927912181824,
1.,0.974927912181824,1.,0.974927912181824,1.,0.974927912181824,1.,0.974927912181824,
1.,0.974927912181824,1.,0.974927912181824,1.,0.974927912181824,1.,0.974927912181824,
1.,0.974927912181824,1.,0.974927912181824,1.,0.974927912181824,1.,0.974927912181824,
1.,0.974927912181824,1.,0.974927912181824,1.,0.974927912181824,1.,0.974927912181824,
1.,0.974927912181824,1.,0.974927912181824,1.,0.974927912181824,1.,0.974927912181824,
1.,0.974927912181824,1.,0.974927912181824,1.,0.974927912181824,1.,0.974927912181824,
1.,0.974927912181824,1.,0.974927912181824,1.,0.974927912181824,1.)))
REPRESENTATION_ITEM('')
SURFACE()
);
#592=CONICAL_SURFACE('',#11051,7.,0.785398163397443);
#597=B_SPLINE_CURVE_WITH_KNOTS('',3,(#14255,#14256,#14257,#14258,#14259,
#14260,#14261,#14262,#14263,#14264,#14265,#14266,#14267,#14268,#14269,#14270,
#14271,#14272,#14273,#14274),.UNSPECIFIED.,.F.,.F.,(4,2,2,2,2,2,2,2,2,4),
(21.0628184025214,21.4115217399649,21.7865786122948,22.1603740098871,22.5335858127541,
22.9068981706492,23.2810500826543,23.656846922793,23.8644254006208,24.0718313053738),
 .UNSPECIFIED.);
#598=B_SPLINE_CURVE_WITH_KNOTS('',3,(#14278,#14279,#14280,#14281,#14282,
#14283,#14284,#14285,#14286,#14287,#14288,#14289,#14290,#14291,#14292,#14293,
#14294,#14295,#14296,#14297),.UNSPECIFIED.,.F.,.F.,(4,2,2,2,2,2,2,2,2,4),
(0.,0.207250737328132,0.414673918623437,0.790189612340599,1.16406160855106,
1.5370946787505,1.91002726915051,2.28354301766879,2.65831929717239,3.00676175776697),
 .UNSPECIFIED.);
#599=B_SPLINE_CURVE_WITH_KNOTS('',3,(#14301,#14302,#14303,#14304,#14305,
#14306,#14307,#14308,#14309,#14310,#14311,#14312,#14313,#14314,#14315,#14316,
#14317,#14318,#14319,#14320,#14321,#14322,#14323,#14324,#14325,#14326,#14327,
#14328,#14329,#14330,#14331,#14332,#14333,#14334,#14335,#14336),
 .UNSPECIFIED.,.F.,.F.,(4,2,2,2,2,2,2,2,2,2,2,2,2,2,2,2,2,4),(3.00676175776697,
3.03504667108494,3.41221154887637,3.78733667813517,4.16097374899924,4.53391428123984,
4.90688520324459,5.28056485337379,5.65563224159108,6.03278211267235,6.40960760837217,
6.78447515598402,7.15800677331664,7.5309813026748,7.90411426490854,8.27808194278114,
8.65356504512735,9.02205372355402),.UNSPECIFIED.);
#600=B_SPLINE_CURVE_WITH_KNOTS('',3,(#14341,#14342,#14343,#14344,#14345,
#14346,#14347,#14348,#14349,#14350,#14351,#14352,#14353,#14354,#14355,#14356,
#14357,#14358,#14359,#14360,#14361,#14362,#14363,#14364,#14365,#14366,#14367,
#14368,#14369,#14370,#14371,#14372,#14373,#14374,#14375,#14376),
 .UNSPECIFIED.,.F.,.F.,(4,2,2,2,2,2,2,2,2,2,2,2,2,2,2,2,2,4),(15.0430228225335,
15.4117873862963,15.7875516106631,16.1617992759669,16.535211600685,16.9084653739098,
17.2822766521976,17.6574248609679,18.0345324837305,18.4119647247325,18.7873129237276,
19.1612723456431,19.5345225088135,19.9077422594671,20.2816590702386,20.6570650535055,
21.034512312453,21.0628184025214),.UNSPECIFIED.);
#601=B_SPLINE_CURVE_WITH_KNOTS('',3,(#14377,#14378,#14379,#14380,#14381,
#14382,#14383,#14384,#14385,#14386,#14387,#14388,#14389,#14390,#14391,#14392,
#14393,#14394,#14395,#14396,#14397,#14398,#14399,#14400,#14401,#14402,#14403,
#14404,#14405,#14406,#14407,#14408,#14409,#14410,#14411,#14412,#14413,#14414),
 .UNSPECIFIED.,.F.,.F.,(4,2,2,2,2,2,2,2,2,2,2,2,2,2,2,2,2,2,4),(9.02205372355402,
9.03126316823583,9.40786592412534,9.78261257335366,10.1561697915982,10.5293045591898,
10.9027222320504,11.2770985056625,11.6531165926403,12.0313420273241,12.4094238490597,
12.7851606240943,13.1592568140597,13.5323951204357,13.9052507331937,14.278528480555,
14.6529947690463,15.0293157755821,15.0385183303645),.UNSPECIFIED.);
#602=B_SPLINE_CURVE_WITH_KNOTS('',3,(#14419,#14420,#14421,#14422,#14423,
#14424,#14425,#14426,#14427,#14428,#14429,#14430,#14431,#14432,#14433,#14434,
#14435,#14436,#14437,#14438,#14439,#14440,#14441,#14442,#14443,#14444,#14445,
#14446,#14447,#14448,#14449,#14450,#14451,#14452,#14453,#14454,#14455,#14456),
 .UNSPECIFIED.,.F.,.F.,(4,2,2,2,2,2,2,2,2,2,2,2,2,2,2,2,2,2,4),(9.02205372357257,
9.03126316825438,9.4078659241447,9.78261257337381,10.1561697916191,10.5293045592115,
10.9027222320728,11.2770985056855,11.653116592664,12.0314814820664,12.409990091939,
12.7862897014773,13.1609462684338,13.5346435169401,13.9080576483678,14.2818945467347,
14.6569217666056,15.0338064827939,15.0430228225335),.UNSPECIFIED.);
#603=B_SPLINE_CURVE_WITH_KNOTS('',3,(#14457,#14458,#14459,#14460,#14461,
#14462,#14463,#14464,#14465,#14466,#14467,#14468,#14469,#14470,#14471,#14472,
#14473,#14474,#14475,#14476,#14477,#14478,#14479,#14480,#14481,#14482,#14483,
#14484,#14485,#14486,#14487,#14488,#14489,#14490,#14491,#14492),
 .UNSPECIFIED.,.F.,.F.,(4,2,2,2,2,2,2,2,2,2,2,2,2,2,2,2,2,4),(15.0385183303645,
15.4067313298554,15.7819335204988,16.1556214204093,16.5284752291602,16.9011707235645,
17.2744228891668,17.6490099855933,18.0255535653001,18.4024212777122,18.7772080652366,
19.1506081528872,19.523300042637,19.8959615653583,20.2693191055988,20.6441635909667,
21.021046298862,21.0493100512724),.UNSPECIFIED.);
#604=B_SPLINE_CURVE_WITH_KNOTS('',3,(#14497,#14498,#14499,#14500,#14501,
#14502,#14503,#14504,#14505,#14506,#14507,#14508,#14509,#14510,#14511,#14512,
#14513,#14514,#14515,#14516,#14517,#14518,#14519,#14520,#14521,#14522,#14523,
#14524,#14525,#14526,#14527,#14528,#14529,#14530,#14531,#14532),
 .UNSPECIFIED.,.F.,.F.,(4,2,2,2,2,2,2,2,2,2,2,2,2,2,2,2,2,4),(3.0067617577732,
3.03504667109116,3.41221154888342,3.78733667814306,4.16097374900799,4.53391428124943,
4.90688520325496,5.28056485338495,5.65563224160295,6.03278211268495,6.40960760838549,
6.78447515599804,7.1580067733314,7.53098130269032,7.90411426492479,8.27808194279812,
8.65356504514509,9.02205372357257),.UNSPECIFIED.);
#605=B_SPLINE_CURVE_WITH_KNOTS('',3,(#14534,#14535,#14536,#14537,#14538,
#14539,#14540,#14541,#14542,#14543,#14544,#14545,#14546,#14547,#14548,#14549,
#14550,#14551,#14552,#14553),.UNSPECIFIED.,.F.,.F.,(4,2,2,2,2,2,2,2,2,4),
(21.0493100512724,21.3974918301899,21.771987726789,22.145224035449,22.5178776222712,
22.8906316137205,23.2642239035516,23.6394586611834,23.8467266621291,24.0538223481184),
 .UNSPECIFIED.);
#606=B_SPLINE_CURVE_WITH_KNOTS('',3,(#14554,#14555,#14556,#14557,#14558,
#14559,#14560,#14561,#14562,#14563,#14564,#14565,#14566,#14567,#14568,#14569,
#14570,#14571,#14572,#14573),.UNSPECIFIED.,.F.,.F.,(4,2,2,2,2,2,2,2,2,4),
(-24.0754558847043,-23.8386618118089,-23.6022771218884,-23.2241633619335,
-22.8481775712266,-22.4739359229648,-22.1006247072007,-21.7274979336969,
-21.3538666435424,-21.0666269184095),.UNSPECIFIED.);
#607=B_SPLINE_CURVE_WITH_KNOTS('',3,(#14579,#14580,#14581,#14582,#14583,
#14584,#14585,#14586,#14587,#14588,#14589,#14590,#14591,#14592,#14593,#14594,
#14595,#14596,#14597,#14598),.UNSPECIFIED.,.F.,.F.,(4,2,2,2,2,2,2,2,2,4),
(-3.0067617577744,-2.658319297179,-2.28354301767456,-1.91002726915535,-1.5370946787543,
-1.16406160855382,-0.790189612342309,-0.414673918624121,-0.207250737328291,
0.),.UNSPECIFIED.);
#608=B_SPLINE_CURVE_WITH_KNOTS('',3,(#14599,#14600,#14601,#14602,#14603,
#14604,#14605,#14606,#14607,#14608,#14609,#14610,#14611,#14612,#14613,#14614,
#14615,#14616,#14617,#14618),.UNSPECIFIED.,.F.,.F.,(4,2,2,2,2,2,2,2,2,4),
(0.,0.207250737328221,0.414673918623899,0.790189612341872,1.16406160855318,
1.53709467875346,1.91002726915431,2.28354301767339,2.65831929717779,3.0067617577732),
 .UNSPECIFIED.);
#609=B_SPLINE_CURVE_WITH_KNOTS('',3,(#14619,#14620,#14621,#14622,#14623,
#14624,#14625,#14626,#14627,#14628,#14629,#14630,#14631,#14632,#14633,#14634,
#14635,#14636,#14637,#14638,#14639,#14640,#14641,#14642,#14643,#14644,#14645,
#14646,#14647,#14648,#14649,#14650,#14651,#14652,#14653,#14654),
 .UNSPECIFIED.,.F.,.F.,(4,2,2,2,2,2,2,2,2,2,2,2,2,2,2,2,2,4),(-21.0666269184095,
-20.9790541549754,-20.6023718836333,-20.2247774596021,-19.8492645538475,
-19.4753390547256,-19.1022007374592,-18.7291148841734,-18.3554001957568,
-17.9803782798469,-17.6033568499733,-17.226173511323,-16.8510033824804,
-16.4772659751798,-16.1041741425224,-15.7310049385523,-15.3570806750968,
-15.0492520168156),.UNSPECIFIED.);
#610=B_SPLINE_CURVE_WITH_KNOTS('',3,(#14659,#14660,#14661,#14662,#14663,
#14664,#14665,#14666,#14667,#14668,#14669,#14670,#14671,#14672,#14673,#14674,
#14675,#14676,#14677,#14678,#14679,#14680,#14681,#14682,#14683,#14684,#14685,
#14686,#14687,#14688,#14689,#14690,#14691,#14692,#14693,#14694),
 .UNSPECIFIED.,.F.,.F.,(4,2,2,2,2,2,2,2,2,2,2,2,2,2,2,2,2,4),(-9.02205372357525,
-8.65356504514781,-8.27808194280083,-7.90411426492742,-7.53098130269283,
-7.15800677333379,-6.7844751560003,-6.40960760838759,-6.03278211268689,
-5.65563224160473,-5.28056485338656,-4.90688520325647,-4.53391428125088,
-4.1609737490094,-3.78733667814442,-3.41221154888473,-3.03504667109241,
-3.0067617577744),.UNSPECIFIED.);
#611=B_SPLINE_CURVE_WITH_KNOTS('',3,(#14695,#14696,#14697,#14698,#14699,
#14700,#14701,#14702,#14703,#14704,#14705,#14706,#14707,#14708,#14709,#14710,
#14711,#14712,#14713,#14714,#14715,#14716,#14717,#14718,#14719,#14720,#14721,
#14722,#14723,#14724,#14725,#14726,#14727,#14728,#14729,#14730),
 .UNSPECIFIED.,.F.,.F.,(4,2,2,2,2,2,2,2,2,2,2,2,2,2,2,2,2,4),(-15.0492520168156,
-14.9817215424698,-14.6042308135452,-14.2273450835583,-13.8523832079359,
-13.4787036832509,-13.1051113288905,-12.731947500807,-12.3585179295024,
-11.9840694865962,-11.6077801414908,-11.2293450863848,-10.8529730003901,
-10.4782699148012,-10.1045515865236,-9.73114186705801,-9.35733692632237,
-9.02845397887332),.UNSPECIFIED.);
#612=B_SPLINE_CURVE_WITH_KNOTS('',3,(#14737,#14738,#14739,#14740,#14741,
#14742,#14743,#14744,#14745,#14746,#14747,#14748,#14749,#14750,#14751,#14752,
#14753,#14754,#14755,#14756,#14757,#14758,#14759,#14760,#14761,#14762,#14763,
#14764,#14765,#14766,#14767,#14768,#14769,#14770,#14771,#14772),
 .UNSPECIFIED.,.F.,.F.,(4,2,2,2,2,2,2,2,2,2,2,2,2,2,2,2,2,4),(-21.062818402533,
-21.0345123124645,-20.6570650535164,-20.2816590702489,-19.9077422594767,
-19.5345225088225,-19.1612723456515,-18.7873129237354,-18.4119647247398,
-18.0345324837374,-17.6574248609745,-17.282276652204,-16.9084653739158,
-16.5352116006907,-16.1617992759723,-15.7875516106682,-15.411787386301,
-15.043022822538),.UNSPECIFIED.);
#613=B_SPLINE_CURVE_WITH_KNOTS('',3,(#14776,#14777,#14778,#14779,#14780,
#14781,#14782,#14783,#14784,#14785,#14786,#14787,#14788,#14789,#14790,#14791,
#14792,#14793,#14794,#14795),.UNSPECIFIED.,.F.,.F.,(4,2,2,2,2,2,2,2,2,4),
(-3.00896219087705,-2.9826900908492,-2.60537804402198,-2.22834522787004,
-1.85329206455909,-1.4795267572371,-1.10637111311519,-0.733142615483747,
-0.359104705713691,0.),.UNSPECIFIED.);
#614=B_SPLINE_CURVE_WITH_KNOTS('',3,(#14798,#14799,#14800,#14801,#14802,
#14803,#14804,#14805,#14806,#14807,#14808,#14809,#14810,#14811,#14812,#14813,
#14814,#14815,#14816,#14817),.UNSPECIFIED.,.F.,.F.,(4,2,2,2,2,2,2,2,2,4),
(-24.0718313053899,-23.8644254006373,-23.6568469228092,-23.2810500826698,
-22.906898170664,-22.5335858127682,-22.1603740099005,-21.7865786123075,
-21.4115217399771,-21.062818402533),.UNSPECIFIED.);
#615=B_SPLINE_CURVE_WITH_KNOTS('',3,(#14851,#14852,#14853,#14854,#14855,
#14856,#14857,#14858,#14859,#14860,#14861,#14862,#14863,#14864,#14865,#14866,
#14867,#14868,#14869,#14870,#14871,#14872,#14873,#14874,#14875,#14876,#14877,
#14878,#14879,#14880,#14881,#14882,#14883,#14884,#14885,#14886,#14887,#14888),
 .UNSPECIFIED.,.F.,.F.,(4,2,2,2,2,2,2,2,2,2,2,2,2,2,2,2,2,2,4),(-15.043022822538,
-15.0338064827984,-14.6569217666099,-14.2818945467388,-13.9080576483717,
-13.5346435169439,-13.1609462684376,-12.7862897014809,-12.4099900919424,
-12.0314814820696,-11.6531165926671,-11.2770985056884,-10.9027222320755,
-10.5293045592142,-10.1561697916218,-9.78261257337648,-9.40786592414737,
-9.03126316825707,-9.02205372357525),.UNSPECIFIED.);
#616=B_SPLINE_CURVE_WITH_KNOTS('',3,(#14889,#14890,#14891,#14892,#14893,
#14894,#14895,#14896,#14897,#14898,#14899,#14900,#14901,#14902,#14903,#14904,
#14905,#14906,#14907,#14908,#14909,#14910,#14911,#14912,#14913,#14914,#14915,
#14916,#14917,#14918,#14919,#14920,#14921,#14922,#14923,#14924),
 .UNSPECIFIED.,.F.,.F.,(4,2,2,2,2,2,2,2,2,2,2,2,2,2,2,2,2,4),(-9.02845397887332,
-8.98237168672322,-8.60557289800359,-8.22751630078672,-7.85170383973507,
-7.47743440461333,-7.10402641355928,-6.73080341422908,-6.35705169861502,
-5.98199451794767,-5.60499798633059,-5.22751545270559,-4.85214443892414,
-4.47818881415784,-4.10496887288142,-3.7318064281611,-3.35797659467942,
-3.00896219087705),.UNSPECIFIED.);
#1322=SHAPE_REPRESENTATION_RELATIONSHIP('SRR','None',#37955,#1334);
#1334=ADVANCED_BREP_SHAPE_REPRESENTATION('',(#1358),#37870);
#1346=STYLED_ITEM('',(#38023),#1358);
#1358=MANIFOLD_SOLID_BREP('Body1',#10820);
#1399=FACE_BOUND('',#2246,.T.);
#1400=FACE_BOUND('',#2248,.T.);
#1401=FACE_BOUND('',#2250,.T.);
#1481=PLANE('',#11066);
#1482=PLANE('',#11067);
#1483=PLANE('',#11068);
#1484=PLANE('',#11069);
#1485=PLANE('',#11072);
#1486=PLANE('',#11074);
#1487=PLANE('',#11075);
#1488=PLANE('',#11076);
#1489=PLANE('',#11077);
#1490=PLANE('',#11078);
#1491=PLANE('',#11079);
#1602=FACE_OUTER_BOUND('',#2233,.T.);
#1603=FACE_OUTER_BOUND('',#2234,.T.);
#1604=FACE_OUTER_BOUND('',#2235,.T.);
#1605=FACE_OUTER_BOUND('',#2236,.T.);
#1606=FACE_OUTER_BOUND('',#2237,.T.);
#1607=FACE_OUTER_BOUND('',#2238,.T.);
#1608=FACE_OUTER_BOUND('',#2239,.T.);
#1609=FACE_OUTER_BOUND('',#2240,.T.);
#1610=FACE_OUTER_BOUND('',#2241,.T.);
#1611=FACE_OUTER_BOUND('',#2242,.T.);
#1612=FACE_OUTER_BOUND('',#2243,.T.);
#1613=FACE_OUTER_BOUND('',#2244,.T.);
#1614=FACE_OUTER_BOUND('',#2245,.T.);
#1615=FACE_OUTER_BOUND('',#2247,.T.);
#1616=FACE_OUTER_BOUND('',#2249,.T.);
#1617=FACE_OUTER_BOUND('',#2251,.T.);
#1618=FACE_OUTER_BOUND('',#2252,.T.);
#1619=FACE_OUTER_BOUND('',#2253,.T.);
#1620=FACE_OUTER_BOUND('',#2254,.T.);
#1621=FACE_OUTER_BOUND('',#2255,.T.);
#1622=FACE_OUTER_BOUND('',#2256,.T.);
#1623=FACE_OUTER_BOUND('',#2257,.T.);
#1624=FACE_OUTER_BOUND('',#2258,.T.);
#1625=FACE_OUTER_BOUND('',#2259,.T.);
#1626=FACE_OUTER_BOUND('',#2260,.T.);
#1627=FACE_OUTER_BOUND('',#2261,.T.);
#1628=FACE_OUTER_BOUND('',#2262,.T.);
#1629=FACE_OUTER_BOUND('',#2263,.T.);
#1630=FACE_OUTER_BOUND('',#2264,.T.);
#2233=EDGE_LOOP('',(#6927,#6928,#6929,#6930,#6931,#6932,#6933,#6934));
#2234=EDGE_LOOP('',(#6935,#6936,#6937,#6938));
#2235=EDGE_LOOP('',(#6939,#6940,#6941,#6942));
#2236=EDGE_LOOP('',(#6943,#6944,#6945,#6946,#6947));
#2237=EDGE_LOOP('',(#6948,#6949,#6950,#6951,#6952));
#2238=EDGE_LOOP('',(#6953,#6954,#6955,#6956));
#2239=EDGE_LOOP('',(#6957,#6958,#6959,#6960,#6961,#6962,#6963,#6964));
#2240=EDGE_LOOP('',(#6965,#6966,#6967,#6968,#6969));
#2241=EDGE_LOOP('',(#6970,#6971,#6972,#6973,#6974,#6975,#6976,#6977));
#2242=EDGE_LOOP('',(#6978,#6979,#6980,#6981));
#2243=EDGE_LOOP('',(#6982,#6983,#6984,#6985,#6986));
#2244=EDGE_LOOP('',(#6987,#6988,#6989,#6990));
#2245=EDGE_LOOP('',(#6991));
#2246=EDGE_LOOP('',(#6992));
#2247=EDGE_LOOP('',(#6993));
#2248=EDGE_LOOP('',(#6994));
#2249=EDGE_LOOP('',(#6995));
#2250=EDGE_LOOP('',(#6996));
#2251=EDGE_LOOP('',(#6997,#6998,#6999,#7000));
#2252=EDGE_LOOP('',(#7001,#7002,#7003,#7004,#7005,#7006,#7007,#7008));
#2253=EDGE_LOOP('',(#7009,#7010,#7011,#7012));
#2254=EDGE_LOOP('',(#7013,#7014,#7015,#7016,#7017,#7018,#7019,#7020));
#2255=EDGE_LOOP('',(#7021,#7022,#7023,#7024));
#2256=EDGE_LOOP('',(#7025,#7026,#7027,#7028,#7029,#7030,#7031,#7032));
#2257=EDGE_LOOP('',(#7033,#7034,#7035,#7036));
#2258=EDGE_LOOP('',(#7037,#7038,#7039,#7040,#7041,#7042,#7043,#7044));
#2259=EDGE_LOOP('',(#7045,#7046,#7047,#7048,#7049));
#2260=EDGE_LOOP('',(#7050,#7051,#7052,#7053));
#2261=EDGE_LOOP('',(#7054,#7055,#7056,#7057));
#2262=EDGE_LOOP('',(#7058,#7059,#7060,#7061));
#2263=EDGE_LOOP('',(#7062,#7063,#7064,#7065));
#2264=EDGE_LOOP('',(#7066));
#2934=LINE('',#14253,#3235);
#2935=LINE('',#14276,#3236);
#2936=LINE('',#14299,#3237);
#2937=LINE('',#14340,#3238);
#2938=LINE('',#14418,#3239);
#2939=LINE('',#14496,#3240);
#2940=LINE('',#14577,#3241);
#2941=LINE('',#14658,#3242);
#2942=LINE('',#14735,#3243);
#2943=LINE('',#14774,#3244);
#2944=LINE('',#14797,#3245);
#2945=LINE('',#14824,#3246);
#2946=LINE('',#14831,#3247);
#2947=LINE('',#14835,#3248);
#2948=LINE('',#14839,#3249);
#2949=LINE('',#14844,#3250);
#2950=LINE('',#14849,#3251);
#2951=LINE('',#14930,#3252);
#2952=LINE('',#14932,#3253);
#2953=LINE('',#15161,#3254);
#2954=LINE('',#16068,#3255);
#2955=LINE('',#16071,#3256);
#2956=LINE('',#16074,#3257);
#2957=LINE('',#17207,#3258);
#2958=LINE('',#17209,#3259);
#2959=LINE('',#17210,#3260);
#2960=LINE('',#17213,#3261);
#2961=LINE('',#17214,#3262);
#2962=LINE('',#17217,#3263);
#2963=LINE('',#17218,#3264);
#2964=LINE('',#17220,#3265);
#3235=VECTOR('',#12111,9.49999999999999);
#3236=VECTOR('',#12112,1000.);
#3237=VECTOR('',#12113,9.49999999999999);
#3238=VECTOR('',#12118,9.49999999999999);
#3239=VECTOR('',#12121,9.49999999999999);
#3240=VECTOR('',#12124,9.49999999999999);
#3241=VECTOR('',#12127,9.49999999999999);
#3242=VECTOR('',#12130,9.49999999999999);
#3243=VECTOR('',#12135,9.49999999999999);
#3244=VECTOR('',#12136,9.49999999999999);
#3245=VECTOR('',#12137,1000.);
#3246=VECTOR('',#12144,7.);
#3247=VECTOR('',#12151,1000.);
#3248=VECTOR('',#12154,7.49999999999999);
#3249=VECTOR('',#12159,1000.);
#3250=VECTOR('',#12164,7.99999999999999);
#3251=VECTOR('',#12171,7.5);
#3252=VECTOR('',#12182,1000.);
#3253=VECTOR('',#12183,1000.);
#3254=VECTOR('',#12186,1000.);
#3255=VECTOR('',#12189,1000.);
#3256=VECTOR('',#12192,1000.);
#3257=VECTOR('',#12195,1000.);
#3258=VECTOR('',#12198,1000.);
#3259=VECTOR('',#12199,1000.);
#3260=VECTOR('',#12200,1000.);
#3261=VECTOR('',#12203,1000.);
#3262=VECTOR('',#12204,1000.);
#3263=VECTOR('',#12207,1000.);
#3264=VECTOR('',#12208,1000.);
#3265=VECTOR('',#12211,1000.);
#3507=CIRCLE('',#11043,9.5);
#3508=CIRCLE('',#11050,9.49999999999999);
#3509=CIRCLE('',#11052,7.5);
#3510=CIRCLE('',#11053,7.5);
#3511=CIRCLE('',#11054,7.);
#3512=CIRCLE('',#11056,7.49999999999999);
#3513=CIRCLE('',#11057,7.49999999999999);
#3514=CIRCLE('',#11058,7.49999999999999);
#3515=CIRCLE('',#11059,7.49999999999999);
#3516=CIRCLE('',#11061,7.99999999999999);
#3517=CIRCLE('',#11062,8.);
#3518=CIRCLE('',#11064,7.5);
#3519=CIRCLE('',#11070,1.);
#3520=CIRCLE('',#11071,1.);
#3521=CIRCLE('',#11073,1.);
#4064=VERTEX_POINT('',#14251);
#4065=VERTEX_POINT('',#14252);
#4066=VERTEX_POINT('',#14254);
#4067=VERTEX_POINT('',#14275);
#4068=VERTEX_POINT('',#14277);
#4069=VERTEX_POINT('',#14298);
#4070=VERTEX_POINT('',#14338);
#4071=VERTEX_POINT('',#14339);
#4072=VERTEX_POINT('',#14416);
#4073=VERTEX_POINT('',#14417);
#4074=VERTEX_POINT('',#14494);
#4075=VERTEX_POINT('',#14495);
#4076=VERTEX_POINT('',#14533);
#4077=VERTEX_POINT('',#14575);
#4078=VERTEX_POINT('',#14576);
#4079=VERTEX_POINT('',#14578);
#4080=VERTEX_POINT('',#14656);
#4081=VERTEX_POINT('',#14657);
#4082=VERTEX_POINT('',#14732);
#4083=VERTEX_POINT('',#14734);
#4084=VERTEX_POINT('',#14736);
#4085=VERTEX_POINT('',#14773);
#4086=VERTEX_POINT('',#14775);
#4087=VERTEX_POINT('',#14796);
#4088=VERTEX_POINT('',#14819);
#4089=VERTEX_POINT('',#14820);
#4090=VERTEX_POINT('',#14823);
#4091=VERTEX_POINT('',#14827);
#4092=VERTEX_POINT('',#14828);
#4093=VERTEX_POINT('',#14830);
#4094=VERTEX_POINT('',#14832);
#4095=VERTEX_POINT('',#14834);
#4096=VERTEX_POINT('',#14837);
#4097=VERTEX_POINT('',#14841);
#4098=VERTEX_POINT('',#14843);
#4099=VERTEX_POINT('',#14847);
#4100=VERTEX_POINT('',#14929);
#4101=VERTEX_POINT('',#14931);
#4102=VERTEX_POINT('',#15160);
#4103=VERTEX_POINT('',#15727);
#4104=VERTEX_POINT('',#16070);
#4105=VERTEX_POINT('',#16072);
#4106=VERTEX_POINT('',#17206);
#4107=VERTEX_POINT('',#17208);
#4108=VERTEX_POINT('',#17212);
#4109=VERTEX_POINT('',#17216);
#5174=EDGE_CURVE('',#4064,#4065,#2934,.T.);
#5175=EDGE_CURVE('',#4065,#4066,#597,.T.);
#5176=EDGE_CURVE('',#4066,#4067,#2935,.T.);
#5177=EDGE_CURVE('',#4068,#4067,#598,.F.);
#5178=EDGE_CURVE('',#4068,#4069,#2936,.T.);
#5179=EDGE_CURVE('',#4069,#4069,#3507,.T.);
#5180=EDGE_CURVE('',#4064,#4068,#599,.F.);
#5181=EDGE_CURVE('',#4070,#4071,#2937,.T.);
#5182=EDGE_CURVE('',#4071,#4065,#600,.T.);
#5183=EDGE_CURVE('',#4070,#4064,#601,.F.);
#5184=EDGE_CURVE('',#4072,#4073,#2938,.T.);
#5185=EDGE_CURVE('',#4073,#4071,#602,.T.);
#5186=EDGE_CURVE('',#4072,#4070,#603,.F.);
#5187=EDGE_CURVE('',#4074,#4075,#2939,.T.);
#5188=EDGE_CURVE('',#4075,#4073,#604,.T.);
#5189=EDGE_CURVE('',#4076,#4072,#605,.F.);
#5190=EDGE_CURVE('',#4076,#4074,#606,.T.);
#5191=EDGE_CURVE('',#4077,#4078,#2940,.T.);
#5192=EDGE_CURVE('',#4079,#4078,#607,.F.);
#5193=EDGE_CURVE('',#4079,#4075,#608,.T.);
#5194=EDGE_CURVE('',#4074,#4077,#609,.T.);
#5195=EDGE_CURVE('',#4080,#4081,#2941,.T.);
#5196=EDGE_CURVE('',#4078,#4081,#610,.F.);
#5197=EDGE_CURVE('',#4077,#4080,#611,.T.);
#5198=EDGE_CURVE('',#4082,#4082,#3508,.T.);
#5199=EDGE_CURVE('',#4082,#4083,#2942,.T.);
#5200=EDGE_CURVE('',#4084,#4083,#612,.F.);
#5201=EDGE_CURVE('',#4085,#4084,#2943,.T.);
#5202=EDGE_CURVE('',#4085,#4086,#613,.T.);
#5203=EDGE_CURVE('',#4087,#4086,#2944,.T.);
#5204=EDGE_CURVE('',#4083,#4087,#614,.F.);
#5205=EDGE_CURVE('',#4088,#4089,#3509,.T.);
#5206=EDGE_CURVE('',#4089,#4088,#3510,.T.);
#5207=EDGE_CURVE('',#4089,#4090,#2945,.T.);
#5208=EDGE_CURVE('',#4090,#4090,#3511,.T.);
#5209=EDGE_CURVE('',#4091,#4092,#3512,.T.);
#5210=EDGE_CURVE('',#4093,#4091,#2946,.T.);
#5211=EDGE_CURVE('',#4094,#4093,#3513,.T.);
#5212=EDGE_CURVE('',#4094,#4095,#2947,.T.);
#5213=EDGE_CURVE('',#4095,#4095,#3514,.T.);
#5214=EDGE_CURVE('',#4096,#4094,#3515,.T.);
#5215=EDGE_CURVE('',#4092,#4096,#2948,.T.);
#5216=EDGE_CURVE('',#4097,#4097,#3516,.T.);
#5217=EDGE_CURVE('',#4097,#4098,#2949,.T.);
#5218=EDGE_CURVE('',#4098,#4098,#3517,.T.);
#5219=EDGE_CURVE('',#4099,#4099,#3518,.T.);
#5220=EDGE_CURVE('',#4099,#4088,#2950,.T.);
#5221=EDGE_CURVE('',#4081,#4084,#615,.F.);
#5222=EDGE_CURVE('',#4080,#4085,#616,.T.);
#5223=EDGE_CURVE('',#4100,#4087,#2951,.T.);
#5224=EDGE_CURVE('',#4086,#4101,#2952,.T.);
#5225=EDGE_CURVE('',#4101,#4100,#3519,.T.);
#5226=EDGE_CURVE('',#4102,#4076,#2953,.T.);
#5227=EDGE_CURVE('',#4102,#4101,#228,.T.);
#5228=EDGE_CURVE('',#4103,#4102,#3520,.T.);
#5229=EDGE_CURVE('',#4103,#4100,#229,.T.);
#5230=EDGE_CURVE('',#4079,#4103,#2954,.T.);
#5231=EDGE_CURVE('',#4104,#4066,#2955,.T.);
#5232=EDGE_CURVE('',#4105,#4104,#3521,.T.);
#5233=EDGE_CURVE('',#4067,#4105,#2956,.T.);
#5234=EDGE_CURVE('',#4102,#4105,#230,.T.);
#5235=EDGE_CURVE('',#4103,#4104,#231,.T.);
#5236=EDGE_CURVE('',#4106,#4093,#2957,.T.);
#5237=EDGE_CURVE('',#4107,#4106,#2958,.T.);
#5238=EDGE_CURVE('',#4096,#4107,#2959,.T.);
#5239=EDGE_CURVE('',#4108,#4091,#2960,.T.);
#5240=EDGE_CURVE('',#4108,#4106,#2961,.T.);
#5241=EDGE_CURVE('',#4109,#4108,#2962,.T.);
#5242=EDGE_CURVE('',#4109,#4107,#2963,.T.);
#5243=EDGE_CURVE('',#4092,#4109,#2964,.T.);
#6927=ORIENTED_EDGE('',*,*,#5174,.T.);
#6928=ORIENTED_EDGE('',*,*,#5175,.T.);
#6929=ORIENTED_EDGE('',*,*,#5176,.T.);
#6930=ORIENTED_EDGE('',*,*,#5177,.F.);
#6931=ORIENTED_EDGE('',*,*,#5178,.T.);
#6932=ORIENTED_EDGE('',*,*,#5179,.T.);
#6933=ORIENTED_EDGE('',*,*,#5178,.F.);
#6934=ORIENTED_EDGE('',*,*,#5180,.F.);
#6935=ORIENTED_EDGE('',*,*,#5181,.T.);
#6936=ORIENTED_EDGE('',*,*,#5182,.T.);
#6937=ORIENTED_EDGE('',*,*,#5174,.F.);
#6938=ORIENTED_EDGE('',*,*,#5183,.F.);
#6939=ORIENTED_EDGE('',*,*,#5184,.T.);
#6940=ORIENTED_EDGE('',*,*,#5185,.T.);
#6941=ORIENTED_EDGE('',*,*,#5181,.F.);
#6942=ORIENTED_EDGE('',*,*,#5186,.F.);
#6943=ORIENTED_EDGE('',*,*,#5187,.T.);
#6944=ORIENTED_EDGE('',*,*,#5188,.T.);
#6945=ORIENTED_EDGE('',*,*,#5184,.F.);
#6946=ORIENTED_EDGE('',*,*,#5189,.F.);
#6947=ORIENTED_EDGE('',*,*,#5190,.T.);
#6948=ORIENTED_EDGE('',*,*,#5191,.T.);
#6949=ORIENTED_EDGE('',*,*,#5192,.F.);
#6950=ORIENTED_EDGE('',*,*,#5193,.T.);
#6951=ORIENTED_EDGE('',*,*,#5187,.F.);
#6952=ORIENTED_EDGE('',*,*,#5194,.T.);
#6953=ORIENTED_EDGE('',*,*,#5195,.T.);
#6954=ORIENTED_EDGE('',*,*,#5196,.F.);
#6955=ORIENTED_EDGE('',*,*,#5191,.F.);
#6956=ORIENTED_EDGE('',*,*,#5197,.T.);
#6957=ORIENTED_EDGE('',*,*,#5198,.F.);
#6958=ORIENTED_EDGE('',*,*,#5199,.T.);
#6959=ORIENTED_EDGE('',*,*,#5200,.F.);
#6960=ORIENTED_EDGE('',*,*,#5201,.F.);
#6961=ORIENTED_EDGE('',*,*,#5202,.T.);
#6962=ORIENTED_EDGE('',*,*,#5203,.F.);
#6963=ORIENTED_EDGE('',*,*,#5204,.F.);
#6964=ORIENTED_EDGE('',*,*,#5199,.F.);
#6965=ORIENTED_EDGE('',*,*,#5205,.F.);
#6966=ORIENTED_EDGE('',*,*,#5206,.F.);
#6967=ORIENTED_EDGE('',*,*,#5207,.T.);
#6968=ORIENTED_EDGE('',*,*,#5208,.F.);
#6969=ORIENTED_EDGE('',*,*,#5207,.F.);
#6970=ORIENTED_EDGE('',*,*,#5209,.F.);
#6971=ORIENTED_EDGE('',*,*,#5210,.F.);
#6972=ORIENTED_EDGE('',*,*,#5211,.F.);
#6973=ORIENTED_EDGE('',*,*,#5212,.T.);
#6974=ORIENTED_EDGE('',*,*,#5213,.T.);
#6975=ORIENTED_EDGE('',*,*,#5212,.F.);
#6976=ORIENTED_EDGE('',*,*,#5214,.F.);
#6977=ORIENTED_EDGE('',*,*,#5215,.F.);
#6978=ORIENTED_EDGE('',*,*,#5216,.F.);
#6979=ORIENTED_EDGE('',*,*,#5217,.T.);
#6980=ORIENTED_EDGE('',*,*,#5218,.T.);
#6981=ORIENTED_EDGE('',*,*,#5217,.F.);
#6982=ORIENTED_EDGE('',*,*,#5219,.F.);
#6983=ORIENTED_EDGE('',*,*,#5220,.T.);
#6984=ORIENTED_EDGE('',*,*,#5205,.T.);
#6985=ORIENTED_EDGE('',*,*,#5206,.T.);
#6986=ORIENTED_EDGE('',*,*,#5220,.F.);
#6987=ORIENTED_EDGE('',*,*,#5201,.T.);
#6988=ORIENTED_EDGE('',*,*,#5221,.F.);
#6989=ORIENTED_EDGE('',*,*,#5195,.F.);
#6990=ORIENTED_EDGE('',*,*,#5222,.T.);
#6991=ORIENTED_EDGE('',*,*,#5179,.F.);
#6992=ORIENTED_EDGE('',*,*,#5219,.T.);
#6993=ORIENTED_EDGE('',*,*,#5198,.T.);
#6994=ORIENTED_EDGE('',*,*,#5218,.F.);
#6995=ORIENTED_EDGE('',*,*,#5216,.T.);
#6996=ORIENTED_EDGE('',*,*,#5213,.F.);
#6997=ORIENTED_EDGE('',*,*,#5223,.T.);
#6998=ORIENTED_EDGE('',*,*,#5203,.T.);
#6999=ORIENTED_EDGE('',*,*,#5224,.T.);
#7000=ORIENTED_EDGE('',*,*,#5225,.T.);
#7001=ORIENTED_EDGE('',*,*,#5226,.F.);
#7002=ORIENTED_EDGE('',*,*,#5227,.T.);
#7003=ORIENTED_EDGE('',*,*,#5224,.F.);
#7004=ORIENTED_EDGE('',*,*,#5202,.F.);
#7005=ORIENTED_EDGE('',*,*,#5222,.F.);
#7006=ORIENTED_EDGE('',*,*,#5197,.F.);
#7007=ORIENTED_EDGE('',*,*,#5194,.F.);
#7008=ORIENTED_EDGE('',*,*,#5190,.F.);
#7009=ORIENTED_EDGE('',*,*,#5228,.F.);
#7010=ORIENTED_EDGE('',*,*,#5229,.T.);
#7011=ORIENTED_EDGE('',*,*,#5225,.F.);
#7012=ORIENTED_EDGE('',*,*,#5227,.F.);
#7013=ORIENTED_EDGE('',*,*,#5230,.F.);
#7014=ORIENTED_EDGE('',*,*,#5192,.T.);
#7015=ORIENTED_EDGE('',*,*,#5196,.T.);
#7016=ORIENTED_EDGE('',*,*,#5221,.T.);
#7017=ORIENTED_EDGE('',*,*,#5200,.T.);
#7018=ORIENTED_EDGE('',*,*,#5204,.T.);
#7019=ORIENTED_EDGE('',*,*,#5223,.F.);
#7020=ORIENTED_EDGE('',*,*,#5229,.F.);
#7021=ORIENTED_EDGE('',*,*,#5176,.F.);
#7022=ORIENTED_EDGE('',*,*,#5231,.F.);
#7023=ORIENTED_EDGE('',*,*,#5232,.F.);
#7024=ORIENTED_EDGE('',*,*,#5233,.F.);
#7025=ORIENTED_EDGE('',*,*,#5226,.T.);
#7026=ORIENTED_EDGE('',*,*,#5189,.T.);
#7027=ORIENTED_EDGE('',*,*,#5186,.T.);
#7028=ORIENTED_EDGE('',*,*,#5183,.T.);
#7029=ORIENTED_EDGE('',*,*,#5180,.T.);
#7030=ORIENTED_EDGE('',*,*,#5177,.T.);
#7031=ORIENTED_EDGE('',*,*,#5233,.T.);
#7032=ORIENTED_EDGE('',*,*,#5234,.F.);
#7033=ORIENTED_EDGE('',*,*,#5228,.T.);
#7034=ORIENTED_EDGE('',*,*,#5234,.T.);
#7035=ORIENTED_EDGE('',*,*,#5232,.T.);
#7036=ORIENTED_EDGE('',*,*,#5235,.F.);
#7037=ORIENTED_EDGE('',*,*,#5230,.T.);
#7038=ORIENTED_EDGE('',*,*,#5235,.T.);
#7039=ORIENTED_EDGE('',*,*,#5231,.T.);
#7040=ORIENTED_EDGE('',*,*,#5175,.F.);
#7041=ORIENTED_EDGE('',*,*,#5182,.F.);
#7042=ORIENTED_EDGE('',*,*,#5185,.F.);
#7043=ORIENTED_EDGE('',*,*,#5188,.F.);
#7044=ORIENTED_EDGE('',*,*,#5193,.F.);
#7045=ORIENTED_EDGE('',*,*,#5236,.F.);
#7046=ORIENTED_EDGE('',*,*,#5237,.F.);
#7047=ORIENTED_EDGE('',*,*,#5238,.F.);
#7048=ORIENTED_EDGE('',*,*,#5214,.T.);
#7049=ORIENTED_EDGE('',*,*,#5211,.T.);
#7050=ORIENTED_EDGE('',*,*,#5210,.T.);
#7051=ORIENTED_EDGE('',*,*,#5239,.F.);
#7052=ORIENTED_EDGE('',*,*,#5240,.T.);
#7053=ORIENTED_EDGE('',*,*,#5236,.T.);
#7054=ORIENTED_EDGE('',*,*,#5237,.T.);
#7055=ORIENTED_EDGE('',*,*,#5240,.F.);
#7056=ORIENTED_EDGE('',*,*,#5241,.F.);
#7057=ORIENTED_EDGE('',*,*,#5242,.T.);
#7058=ORIENTED_EDGE('',*,*,#5215,.T.);
#7059=ORIENTED_EDGE('',*,*,#5238,.T.);
#7060=ORIENTED_EDGE('',*,*,#5242,.F.);
#7061=ORIENTED_EDGE('',*,*,#5243,.F.);
#7062=ORIENTED_EDGE('',*,*,#5209,.T.);
#7063=ORIENTED_EDGE('',*,*,#5243,.T.);
#7064=ORIENTED_EDGE('',*,*,#5241,.T.);
#7065=ORIENTED_EDGE('',*,*,#5239,.T.);
#7066=ORIENTED_EDGE('',*,*,#5208,.T.);
#10050=CYLINDRICAL_SURFACE('',#11042,9.49999999999999);
#10051=CYLINDRICAL_SURFACE('',#11044,9.49999999999999);
#10052=CYLINDRICAL_SURFACE('',#11045,9.49999999999999);
#10053=CYLINDRICAL_SURFACE('',#11046,9.49999999999999);
#10054=CYLINDRICAL_SURFACE('',#11047,9.49999999999999);
#10055=CYLINDRICAL_SURFACE('',#11048,9.49999999999999);
#10056=CYLINDRICAL_SURFACE('',#11049,9.49999999999999);
#10057=CYLINDRICAL_SURFACE('',#11055,7.49999999999999);
#10058=CYLINDRICAL_SURFACE('',#11060,7.99999999999999);
#10059=CYLINDRICAL_SURFACE('',#11063,7.5);
#10060=CYLINDRICAL_SURFACE('',#11065,9.49999999999999);
#10247=ADVANCED_FACE('',(#1602),#10050,.T.);
#10248=ADVANCED_FACE('',(#1603),#10051,.T.);
#10249=ADVANCED_FACE('',(#1604),#10052,.T.);
#10250=ADVANCED_FACE('',(#1605),#10053,.T.);
#10251=ADVANCED_FACE('',(#1606),#10054,.T.);
#10252=ADVANCED_FACE('',(#1607),#10055,.T.);
#10253=ADVANCED_FACE('',(#1608),#10056,.T.);
#10254=ADVANCED_FACE('',(#1609),#592,.T.);
#10255=ADVANCED_FACE('',(#1610),#10057,.T.);
#10256=ADVANCED_FACE('',(#1611),#10058,.T.);
#10257=ADVANCED_FACE('',(#1612),#10059,.T.);
#10258=ADVANCED_FACE('',(#1613),#10060,.T.);
#10259=ADVANCED_FACE('',(#1614,#1399),#1481,.T.);
#10260=ADVANCED_FACE('',(#1615,#1400),#1482,.T.);
#10261=ADVANCED_FACE('',(#1616,#1401),#1483,.T.);
#10262=ADVANCED_FACE('',(#1617),#1484,.T.);
#10263=ADVANCED_FACE('',(#1618),#322,.F.);
#10264=ADVANCED_FACE('',(#1619),#323,.F.);
#10265=ADVANCED_FACE('',(#1620),#324,.F.);
#10266=ADVANCED_FACE('',(#1621),#1485,.F.);
#10267=ADVANCED_FACE('',(#1622),#325,.T.);
#10268=ADVANCED_FACE('',(#1623),#326,.T.);
#10269=ADVANCED_FACE('',(#1624),#327,.T.);
#10270=ADVANCED_FACE('',(#1625),#1486,.T.);
#10271=ADVANCED_FACE('',(#1626),#1487,.F.);
#10272=ADVANCED_FACE('',(#1627),#1488,.F.);
#10273=ADVANCED_FACE('',(#1628),#1489,.F.);
#10274=ADVANCED_FACE('',(#1629),#1490,.F.);
#10275=ADVANCED_FACE('',(#1630),#1491,.T.);
#10820=CLOSED_SHELL('',(#10247,#10248,#10249,#10250,#10251,#10252,#10253,
#10254,#10255,#10256,#10257,#10258,#10259,#10260,#10261,#10262,#10263,#10264,
#10265,#10266,#10267,#10268,#10269,#10270,#10271,#10272,#10273,#10274,#10275));
#11041=AXIS2_PLACEMENT_3D('',#14249,#12107,#12108);
#11042=AXIS2_PLACEMENT_3D('',#14250,#12109,#12110);
#11043=AXIS2_PLACEMENT_3D('',#14300,#12114,#12115);
#11044=AXIS2_PLACEMENT_3D('',#14337,#12116,#12117);
#11045=AXIS2_PLACEMENT_3D('',#14415,#12119,#12120);
#11046=AXIS2_PLACEMENT_3D('',#14493,#12122,#12123);
#11047=AXIS2_PLACEMENT_3D('',#14574,#12125,#12126);
#11048=AXIS2_PLACEMENT_3D('',#14655,#12128,#12129);
#11049=AXIS2_PLACEMENT_3D('',#14731,#12131,#12132);
#11050=AXIS2_PLACEMENT_3D('',#14733,#12133,#12134);
#11051=AXIS2_PLACEMENT_3D('',#14818,#12138,#12139);
#11052=AXIS2_PLACEMENT_3D('',#14821,#12140,#12141);
#11053=AXIS2_PLACEMENT_3D('',#14822,#12142,#12143);
#11054=AXIS2_PLACEMENT_3D('',#14825,#12145,#12146);
#11055=AXIS2_PLACEMENT_3D('',#14826,#12147,#12148);
#11056=AXIS2_PLACEMENT_3D('',#14829,#12149,#12150);
#11057=AXIS2_PLACEMENT_3D('',#14833,#12152,#12153);
#11058=AXIS2_PLACEMENT_3D('',#14836,#12155,#12156);
#11059=AXIS2_PLACEMENT_3D('',#14838,#12157,#12158);
#11060=AXIS2_PLACEMENT_3D('',#14840,#12160,#12161);
#11061=AXIS2_PLACEMENT_3D('',#14842,#12162,#12163);
#11062=AXIS2_PLACEMENT_3D('',#14845,#12165,#12166);
#11063=AXIS2_PLACEMENT_3D('',#14846,#12167,#12168);
#11064=AXIS2_PLACEMENT_3D('',#14848,#12169,#12170);
#11065=AXIS2_PLACEMENT_3D('',#14850,#12172,#12173);
#11066=AXIS2_PLACEMENT_3D('',#14925,#12174,#12175);
#11067=AXIS2_PLACEMENT_3D('',#14926,#12176,#12177);
#11068=AXIS2_PLACEMENT_3D('',#14927,#12178,#12179);
#11069=AXIS2_PLACEMENT_3D('',#14928,#12180,#12181);
#11070=AXIS2_PLACEMENT_3D('',#14933,#12184,#12185);
#11071=AXIS2_PLACEMENT_3D('',#15728,#12187,#12188);
#11072=AXIS2_PLACEMENT_3D('',#16069,#12190,#12191);
#11073=AXIS2_PLACEMENT_3D('',#16073,#12193,#12194);
#11074=AXIS2_PLACEMENT_3D('',#17205,#12196,#12197);
#11075=AXIS2_PLACEMENT_3D('',#17211,#12201,#12202);
#11076=AXIS2_PLACEMENT_3D('',#17215,#12205,#12206);
#11077=AXIS2_PLACEMENT_3D('',#17219,#12209,#12210);
#11078=AXIS2_PLACEMENT_3D('',#17221,#12212,#12213);
#11079=AXIS2_PLACEMENT_3D('',#17222,#12214,#12215);
#12107=DIRECTION('axis',(0.,0.,1.));
#12108=DIRECTION('refdir',(1.,0.,0.));
#12109=DIRECTION('center_axis',(1.,1.34590614515444E-16,0.));
#12110=DIRECTION('ref_axis',(-1.34590614515444E-16,1.,0.));
#12111=DIRECTION('',(-1.,-1.34590614515444E-16,0.));
#12112=DIRECTION('',(-1.,-1.34590614515444E-16,0.));
#12113=DIRECTION('',(-1.,-1.34590614515444E-16,0.));
#12114=DIRECTION('center_axis',(1.,1.34590614515444E-16,0.));
#12115=DIRECTION('ref_axis',(-1.34590614515444E-16,1.,0.));
#12116=DIRECTION('center_axis',(1.,1.34590614515444E-16,0.));
#12117=DIRECTION('ref_axis',(-1.34590614515444E-16,1.,0.));
#12118=DIRECTION('',(-1.,-1.34590614515444E-16,0.));
#12119=DIRECTION('center_axis',(1.,1.34590614515444E-16,0.));
#12120=DIRECTION('ref_axis',(-1.34590614515444E-16,1.,0.));
#12121=DIRECTION('',(-1.,-1.34590614515444E-16,0.));
#12122=DIRECTION('center_axis',(1.,1.34590614515444E-16,0.));
#12123=DIRECTION('ref_axis',(-1.34590614515444E-16,1.,0.));
#12124=DIRECTION('',(-1.,-1.34590614515444E-16,0.));
#12125=DIRECTION('center_axis',(1.,1.34590614515444E-16,0.));
#12126=DIRECTION('ref_axis',(-1.34590614515444E-16,1.,0.));
#12127=DIRECTION('',(-1.,-1.34590614515444E-16,0.));
#12128=DIRECTION('center_axis',(1.,1.34590614515444E-16,0.));
#12129=DIRECTION('ref_axis',(-1.34590614515444E-16,1.,0.));
#12130=DIRECTION('',(-1.,-1.34590614515444E-16,0.));
#12131=DIRECTION('center_axis',(1.,1.34590614515444E-16,0.));
#12132=DIRECTION('ref_axis',(-1.34590614515444E-16,1.,0.));
#12133=DIRECTION('center_axis',(1.,1.34590614515444E-16,0.));
#12134=DIRECTION('ref_axis',(-1.34590614515444E-16,1.,0.));
#12135=DIRECTION('',(-1.,-1.34590614515444E-16,0.));
#12136=DIRECTION('',(-1.,-1.34590614515444E-16,0.));
#12137=DIRECTION('',(-1.,-1.34590614515444E-16,0.));
#12138=DIRECTION('center_axis',(1.,2.36658271566304E-30,0.));
#12139=DIRECTION('ref_axis',(0.,0.,-1.));
#12140=DIRECTION('center_axis',(1.,2.36658271566304E-30,0.));
#12141=DIRECTION('ref_axis',(8.21073318940323E-45,-3.46944695195362E-15,
1.));
#12142=DIRECTION('center_axis',(1.,2.36658271566304E-30,0.));
#12143=DIRECTION('ref_axis',(8.21073318940323E-45,-3.46944695195362E-15,
1.));
#12144=DIRECTION('',(-0.707106781186551,8.65956056235472E-17,-0.707106781186544));
#12145=DIRECTION('center_axis',(-1.,-1.34590614515444E-16,0.));
#12146=DIRECTION('ref_axis',(1.34590614515444E-16,-1.,0.));
#12147=DIRECTION('center_axis',(1.,1.34590614515444E-16,0.));
#12148=DIRECTION('ref_axis',(-1.34590614515444E-16,1.,0.));
#12149=DIRECTION('center_axis',(1.,2.36658271566304E-30,0.));
#12150=DIRECTION('ref_axis',(-1.25897908904183E-44,5.31981865966221E-15,
1.));
#12151=DIRECTION('',(-1.,-1.34590614515444E-16,0.));
#12152=DIRECTION('center_axis',(1.,1.34590614515444E-16,0.));
#12153=DIRECTION('ref_axis',(-1.34590614515444E-16,1.,0.));
#12154=DIRECTION('',(-1.,-1.34590614515444E-16,0.));
#12155=DIRECTION('center_axis',(1.,1.34590614515444E-16,0.));
#12156=DIRECTION('ref_axis',(-1.34590614515444E-16,1.,0.));
#12157=DIRECTION('center_axis',(1.,1.34590614515444E-16,0.));
#12158=DIRECTION('ref_axis',(-1.34590614515444E-16,1.,0.));
#12159=DIRECTION('',(1.,1.34590614515444E-16,0.));
#12160=DIRECTION('center_axis',(1.,1.34590614515444E-16,0.));
#12161=DIRECTION('ref_axis',(-1.34590614515444E-16,1.,0.));
#12162=DIRECTION('center_axis',(1.,1.34590614515444E-16,0.));
#12163=DIRECTION('ref_axis',(-1.34590614515444E-16,1.,0.));
#12164=DIRECTION('',(-1.,-1.34590614515444E-16,0.));
#12165=DIRECTION('center_axis',(1.,1.34590614515444E-16,0.));
#12166=DIRECTION('ref_axis',(-1.34590614515444E-16,1.,0.));
#12167=DIRECTION('center_axis',(1.,1.34590614515444E-16,0.));
#12168=DIRECTION('ref_axis',(-1.34590614515444E-16,1.,0.));
#12169=DIRECTION('center_axis',(1.,1.34590614515444E-16,0.));
#12170=DIRECTION('ref_axis',(-1.34590614515444E-16,1.,0.));
#12171=DIRECTION('',(-1.,-1.34590614515444E-16,0.));
#12172=DIRECTION('center_axis',(1.,1.34590614515444E-16,0.));
#12173=DIRECTION('ref_axis',(-1.34590614515444E-16,1.,0.));
#12174=DIRECTION('center_axis',(-1.,-1.3459061451544E-16,0.));
#12175=DIRECTION('ref_axis',(1.3459061451544E-16,-1.,0.));
#12176=DIRECTION('center_axis',(1.,1.3459061451544E-16,0.));
#12177=DIRECTION('ref_axis',(-1.3459061451544E-16,1.,0.));
#12178=DIRECTION('center_axis',(1.,1.3459061451544E-16,0.));
#12179=DIRECTION('ref_axis',(-1.3459061451544E-16,1.,0.));
#12180=DIRECTION('center_axis',(0.,0.,-1.));
#12181=DIRECTION('ref_axis',(-1.,-2.36658271566304E-30,0.));
#12182=DIRECTION('',(0.241125309054894,-0.970493990364279,0.));
#12183=DIRECTION('',(0.241125309054894,0.970493990364279,5.55111512312579E-17));
#12184=DIRECTION('center_axis',(0.,0.,-1.));
#12185=DIRECTION('ref_axis',(0.970493990364279,0.241125309054894,0.));
#12186=DIRECTION('',(-0.241125309054894,-0.970493990364279,-5.55111512312578E-17));
#12187=DIRECTION('center_axis',(0.,0.,1.));
#12188=DIRECTION('ref_axis',(0.970493990364279,0.241125309054895,0.));
#12189=DIRECTION('',(-0.241125309054895,0.970493990364279,-5.55111512312579E-17));
#12190=DIRECTION('center_axis',(0.,0.,-1.));
#12191=DIRECTION('ref_axis',(-1.,-2.36658271566304E-30,0.));
#12192=DIRECTION('',(0.241125309054894,-0.970493990364279,0.));
#12193=DIRECTION('center_axis',(0.,0.,-1.));
#12194=DIRECTION('ref_axis',(0.970493990364278,0.241125309054898,0.));
#12195=DIRECTION('',(0.241125309054894,0.970493990364279,5.55111512312579E-17));
#12196=DIRECTION('center_axis',(1.,1.3459061451544E-16,0.));
#12197=DIRECTION('ref_axis',(-1.3459061451544E-16,1.,0.));
#12198=DIRECTION('',(1.57772181044202E-30,1.,0.));
#12199=DIRECTION('',(3.94430452610506E-31,0.,-1.));
#12200=DIRECTION('',(-1.57772181044202E-30,-1.,0.));
#12201=DIRECTION('center_axis',(0.,0.,-1.));
#12202=DIRECTION('ref_axis',(-1.,-2.36658271566304E-30,0.));
#12203=DIRECTION('',(1.57772181044202E-30,1.,0.));
#12204=DIRECTION('',(1.,1.34590614515444E-16,0.));
#12205=DIRECTION('center_axis',(1.34590614515444E-16,-1.,0.));
#12206=DIRECTION('ref_axis',(1.,1.34590614515444E-16,0.));
#12207=DIRECTION('',(3.94430452610506E-31,0.,-1.));
#12208=DIRECTION('',(1.,1.34590614515444E-16,0.));
#12209=DIRECTION('center_axis',(0.,0.,1.));
#12210=DIRECTION('ref_axis',(1.,2.36658271566304E-30,0.));
#12211=DIRECTION('',(-1.57772181044202E-30,-1.,0.));
#12212=DIRECTION('center_axis',(-1.,-2.36658271566304E-30,0.));
#12213=DIRECTION('ref_axis',(0.,0.,1.));
#12214=DIRECTION('center_axis',(-1.,-1.3459061451544E-16,0.));
#12215=DIRECTION('ref_axis',(1.3459061451544E-16,-1.,0.));
#14249=CARTESIAN_POINT('',(0.,0.,0.));
#14250=CARTESIAN_POINT('Origin',(78.0000000000001,-11.7,-3.46944695195361E-15));
#14251=CARTESIAN_POINT('',(-16.9,-21.2,-5.09198826713469E-15));
#14252=CARTESIAN_POINT('',(-19.1,-21.2,2.01131938556989E-13));
#14253=CARTESIAN_POINT('',(78.0000000000001,-21.2,-4.6328614111436E-15));
#14254=CARTESIAN_POINT('',(-22.1,-2.20000000000001,-2.08166817117217E-14));
#14255=CARTESIAN_POINT('Ctrl Pts',(-19.1,-21.2,4.05231403988182E-13));
#14256=CARTESIAN_POINT('Ctrl Pts',(-19.2141053600769,-21.2,-1.15460863648497));
#14257=CARTESIAN_POINT('Ctrl Pts',(-19.332091158415,-20.9895203441917,-2.30044202055597));
#14258=CARTESIAN_POINT('Ctrl Pts',(-19.5730265024687,-20.1352887413494,
-4.54344435292798));
#14259=CARTESIAN_POINT('Ctrl Pts',(-19.6962929725925,-19.4685757291998,
-5.60768898329886));
#14260=CARTESIAN_POINT('Ctrl Pts',(-19.947172704971,-17.7660153225662,-7.4155252102245));
#14261=CARTESIAN_POINT('Ctrl Pts',(-20.0685650512849,-16.7477137680798,
-8.14290619632582));
#14262=CARTESIAN_POINT('Ctrl Pts',(-20.319586856915,-14.4912108845094,-9.16464314019048));
#14263=CARTESIAN_POINT('Ctrl Pts',(-20.4403562347154,-13.274900868981,-9.44993444082396));
#14264=CARTESIAN_POINT('Ctrl Pts',(-20.6911293307758,-10.8010005184202,
-9.53803958026904));
#14265=CARTESIAN_POINT('Ctrl Pts',(-20.8125911601839,-9.5670200122243,-9.33986229220506));
#14266=CARTESIAN_POINT('Ctrl Pts',(-21.0627326460083,-7.24203907542784,
-8.48033707933769));
#14267=CARTESIAN_POINT('Ctrl Pts',(-21.1861739757011,-6.17366151377902,
-7.82617419694351));
#14268=CARTESIAN_POINT('Ctrl Pts',(-21.4353260823092,-4.34505010391497,
-6.14065935137859));
#14269=CARTESIAN_POINT('Ctrl Pts',(-21.5619357157688,-3.60400801504437,
-5.12410600030777));
#14270=CARTESIAN_POINT('Ctrl Pts',(-21.7536591008347,-2.79107732111429,
-3.36964268186332));
#14271=CARTESIAN_POINT('Ctrl Pts',(-21.8232454680744,-2.57052382279367,
-2.71585246112488));
#14272=CARTESIAN_POINT('Ctrl Pts',(-21.9626425064765,-2.27462673223657,
-1.37285912097139));
#14273=CARTESIAN_POINT('Ctrl Pts',(-22.032058430158,-2.20000000000001,-0.687486751394685));
#14274=CARTESIAN_POINT('Ctrl Pts',(-22.1,-2.20000000000001,-2.52575738102223E-14));
#14275=CARTESIAN_POINT('',(-25.9,-2.20000000000001,-2.08166817117217E-14));
#14276=CARTESIAN_POINT('',(78.0000000000001,-2.19999999999999,-1.38777878078145E-14));
#14277=CARTESIAN_POINT('',(-22.9,-21.2,1.91278709213441E-13));
#14278=CARTESIAN_POINT('Ctrl Pts',(-25.9,-2.20000000000001,-1.346145417358E-14));
#14279=CARTESIAN_POINT('Ctrl Pts',(-25.8320584301579,-2.20000000000001,
-0.687486751394945));
#14280=CARTESIAN_POINT('Ctrl Pts',(-25.7626425064764,-2.27462673223674,
-1.3728591209719));
#14281=CARTESIAN_POINT('Ctrl Pts',(-25.6232454680743,-2.57052382279374,
-2.71585246112496));
#14282=CARTESIAN_POINT('Ctrl Pts',(-25.5536591008347,-2.79107732111439,
-3.36964268186342));
#14283=CARTESIAN_POINT('Ctrl Pts',(-25.3619357157688,-3.60400801504449,
-5.12410600030786));
#14284=CARTESIAN_POINT('Ctrl Pts',(-25.2353260823091,-4.34505010391509,
-6.14065935137866));
#14285=CARTESIAN_POINT('Ctrl Pts',(-24.986173975701,-6.1736615137792,-7.82617419694359));
#14286=CARTESIAN_POINT('Ctrl Pts',(-24.8627326460082,-7.24203907542804,
-8.48033707933774));
#14287=CARTESIAN_POINT('Ctrl Pts',(-24.6125911601838,-9.5670200122245,-9.33986229220506));
#14288=CARTESIAN_POINT('Ctrl Pts',(-24.4911293307757,-10.8010005184203,
-9.53803958026902));
#14289=CARTESIAN_POINT('Ctrl Pts',(-24.2403562347153,-13.2749008689812,
-9.44993444082388));
#14290=CARTESIAN_POINT('Ctrl Pts',(-24.1195868569149,-14.4912108845096,
-9.16464314019041));
#14291=CARTESIAN_POINT('Ctrl Pts',(-23.8685650512848,-16.7477137680801,
-8.14290619632563));
#14292=CARTESIAN_POINT('Ctrl Pts',(-23.747172704971,-17.7660153225664,-7.41552521022427));
#14293=CARTESIAN_POINT('Ctrl Pts',(-23.4962929725924,-19.4685757292,-5.60768898329859));
#14294=CARTESIAN_POINT('Ctrl Pts',(-23.3730265024686,-20.1352887413495,
-4.54344435292771));
#14295=CARTESIAN_POINT('Ctrl Pts',(-23.132091158415,-20.9895203441917,-2.3004420205559));
#14296=CARTESIAN_POINT('Ctrl Pts',(-23.0141053600769,-21.2,-1.15460863648495));
#14297=CARTESIAN_POINT('Ctrl Pts',(-22.9,-21.2,3.88855614374961E-13));
#14298=CARTESIAN_POINT('',(-28.,-21.2,-4.6328614111436E-15));
#14299=CARTESIAN_POINT('',(78.0000000000001,-21.2,-4.6328614111436E-15));
#14300=CARTESIAN_POINT('Origin',(-28.,-11.7,-1.38777878078145E-14));
#14301=CARTESIAN_POINT('Ctrl Pts',(-22.9,-21.2,3.87190279838026E-13));
#14302=CARTESIAN_POINT('Ctrl Pts',(-22.8907374657687,-21.2,0.0937256760946458));
#14303=CARTESIAN_POINT('Ctrl Pts',(-22.8814385325659,-21.1986129794597,
0.187503087496975));
#14304=CARTESIAN_POINT('Ctrl Pts',(-22.7476627637501,-21.158782162885,1.53206141455917));
#14305=CARTESIAN_POINT('Ctrl Pts',(-22.6195857027287,-20.8749735642952,
2.76326935456493));
#14306=CARTESIAN_POINT('Ctrl Pts',(-22.3715836109607,-19.8492914847688,
5.03864619904501));
#14307=CARTESIAN_POINT('Ctrl Pts',(-22.2456483173604,-19.1196837186759,
6.06203761529605));
#14308=CARTESIAN_POINT('Ctrl Pts',(-21.9962859433281,-17.3106672228239,
7.76583202293418));
#14309=CARTESIAN_POINT('Ctrl Pts',(-21.8733077828502,-16.2500729662692,
8.43116573925417));
#14310=CARTESIAN_POINT('Ctrl Pts',(-21.6230205555366,-13.9355883064945,
9.3158003799263));
#14311=CARTESIAN_POINT('Ctrl Pts',(-21.5017872572193,-12.7041409356645,
9.52751127093411));
#14312=CARTESIAN_POINT('Ctrl Pts',(-21.2509382405826,-10.2294916214254,
9.46676421981238));
#14313=CARTESIAN_POINT('Ctrl Pts',(-21.1301518730001,-9.00991703997751,
9.19486269390215));
#14314=CARTESIAN_POINT('Ctrl Pts',(-20.8791269559889,-6.7415612104141,8.19766790339056));
#14315=CARTESIAN_POINT('Ctrl Pts',(-20.7574769583156,-5.7148544442386,7.48105206827987));
#14316=CARTESIAN_POINT('Ctrl Pts',(-20.5066661962114,-3.99170948168168,
5.69050173900247));
#14317=CARTESIAN_POINT('Ctrl Pts',(-20.3829213282128,-3.31314727879795,
4.63251285108534));
#14318=CARTESIAN_POINT('Ctrl Pts',(-20.1327007105934,-2.40024227986376,
2.30894656775527));
#14319=CARTESIAN_POINT('Ctrl Pts',(-20.005768200205,-2.17734057865521,1.0650747678804));
#14320=CARTESIAN_POINT('Ctrl Pts',(-19.7575217818351,-2.22627476101522,
-1.43571070081335));
#14321=CARTESIAN_POINT('Ctrl Pts',(-19.6295778173592,-2.49719213060869,
-2.66851420318476));
#14322=CARTESIAN_POINT('Ctrl Pts',(-19.3812911783324,-3.49816598006772,
-4.95240981504498));
#14323=CARTESIAN_POINT('Ctrl Pts',(-19.2559908218536,-4.21629480933593,
-5.98259204016963));
#14324=CARTESIAN_POINT('Ctrl Pts',(-19.0064304834418,-6.00563654506256,
-7.70457444607862));
#14325=CARTESIAN_POINT('Ctrl Pts',(-18.8838716533655,-7.05840175783298,
-8.38103212678982));
#14326=CARTESIAN_POINT('Ctrl Pts',(-18.6334518017468,-9.36229409907318,
-9.29067738573382));
#14327=CARTESIAN_POINT('Ctrl Pts',(-18.512401104484,-10.5911524555273,-9.5158718365491));
#14328=CARTESIAN_POINT('Ctrl Pts',(-18.2614900330185,-13.0664139465303,
-9.4823822891556));
#14329=CARTESIAN_POINT('Ctrl Pts',(-18.1406407820112,-14.2891812567478,
-9.22382157527658));
#14330=CARTESIAN_POINT('Ctrl Pts',(-17.889626499178,-16.5692015069562,-8.25108999017966));
#14331=CARTESIAN_POINT('Ctrl Pts',(-17.7676770718268,-17.6042062462676,
-7.54520943878782));
#14332=CARTESIAN_POINT('Ctrl Pts',(-17.5169480501853,-19.3476995003355,
-5.77191772591639));
#14333=CARTESIAN_POINT('Ctrl Pts',(-17.392688674322,-20.0379796864886,-4.72019166334915));
#14334=CARTESIAN_POINT('Ctrl Pts',(-17.1456751427851,-20.9644157250574,
-2.43216559502745));
#14335=CARTESIAN_POINT('Ctrl Pts',(-17.0207145116956,-21.2,-1.22148528043644));
#14336=CARTESIAN_POINT('Ctrl Pts',(-16.9,-21.2,-5.55111512312578E-15));
#14337=CARTESIAN_POINT('Origin',(78.0000000000001,-11.7,-3.46944695195361E-15));
#14338=CARTESIAN_POINT('',(-10.9,-21.2,-1.23573508489533E-14));
#14339=CARTESIAN_POINT('',(-13.1,-21.2,7.39802075989836E-15));
#14340=CARTESIAN_POINT('',(78.0000000000001,-21.2,-4.6328614111436E-15));
#14341=CARTESIAN_POINT('Ctrl Pts',(-13.1,-21.2,2.02615701994091E-14));
#14342=CARTESIAN_POINT('Ctrl Pts',(-13.2207145116956,-21.2,-1.22148528043635));
#14343=CARTESIAN_POINT('Ctrl Pts',(-13.3456751427851,-20.9644157250575,
-2.43216559502735));
#14344=CARTESIAN_POINT('Ctrl Pts',(-13.592688674322,-20.0379796864885,-4.72019166334929));
#14345=CARTESIAN_POINT('Ctrl Pts',(-13.7169480501853,-19.3476995003353,
-5.77191772591653));
#14346=CARTESIAN_POINT('Ctrl Pts',(-13.9676770718269,-17.6042062462674,
-7.5452094387879));
#14347=CARTESIAN_POINT('Ctrl Pts',(-14.089626499178,-16.569201506956,-8.25108999017973));
#14348=CARTESIAN_POINT('Ctrl Pts',(-14.3406407820113,-14.2891812567476,
-9.22382157527662));
#14349=CARTESIAN_POINT('Ctrl Pts',(-14.4614900330186,-13.0664139465301,
-9.4823822891556));
#14350=CARTESIAN_POINT('Ctrl Pts',(-14.7124011044841,-10.591152455527,-9.51587183654904));
#14351=CARTESIAN_POINT('Ctrl Pts',(-14.8334518017469,-9.36229409907295,
-9.29067738573371));
#14352=CARTESIAN_POINT('Ctrl Pts',(-15.0838716533656,-7.05840175783286,
-8.38103212678968));
#14353=CARTESIAN_POINT('Ctrl Pts',(-15.2064304834419,-6.0056365450624,-7.70457444607847));
#14354=CARTESIAN_POINT('Ctrl Pts',(-15.4559908218536,-4.21629480933576,
-5.98259204016936));
#14355=CARTESIAN_POINT('Ctrl Pts',(-15.5812911783325,-3.49816598006762,
-4.95240981504472));
#14356=CARTESIAN_POINT('Ctrl Pts',(-15.8295778173592,-2.49719213060864,
-2.66851420318443));
#14357=CARTESIAN_POINT('Ctrl Pts',(-15.9575217818352,-2.22627476101525,
-1.43571070081306));
#14358=CARTESIAN_POINT('Ctrl Pts',(-16.2057682002051,-2.1773405786553,1.0650747678805));
#14359=CARTESIAN_POINT('Ctrl Pts',(-16.3327007105934,-2.40024227986371,
2.30894656775527));
#14360=CARTESIAN_POINT('Ctrl Pts',(-16.5829213282129,-3.31314727879807,
4.63251285108554));
#14361=CARTESIAN_POINT('Ctrl Pts',(-16.7066661962114,-3.99170948168173,
5.69050173900263));
#14362=CARTESIAN_POINT('Ctrl Pts',(-16.9574769583157,-5.71485444423879,
7.48105206828005));
#14363=CARTESIAN_POINT('Ctrl Pts',(-17.079126955989,-6.74156121041422,8.19766790339073));
#14364=CARTESIAN_POINT('Ctrl Pts',(-17.3301518730003,-9.00991703997782,
9.19486269390231));
#14365=CARTESIAN_POINT('Ctrl Pts',(-17.4509382405827,-10.2294916214257,
9.46676421981248));
#14366=CARTESIAN_POINT('Ctrl Pts',(-17.7017872572195,-12.7041409356649,
9.52751127093413));
#14367=CARTESIAN_POINT('Ctrl Pts',(-17.8230205555367,-13.9355883064948,
9.31580037992625));
#14368=CARTESIAN_POINT('Ctrl Pts',(-18.0733077828503,-16.2500729662695,
8.43116573925405));
#14369=CARTESIAN_POINT('Ctrl Pts',(-18.1962859433283,-17.3106672228242,
7.76583202293403));
#14370=CARTESIAN_POINT('Ctrl Pts',(-18.4456483173605,-19.1196837186761,
6.06203761529587));
#14371=CARTESIAN_POINT('Ctrl Pts',(-18.5715836109608,-19.849291484769,5.0386461990448));
#14372=CARTESIAN_POINT('Ctrl Pts',(-18.8195857027288,-20.8749735642953,
2.76326935456469));
#14373=CARTESIAN_POINT('Ctrl Pts',(-18.9476627637502,-21.1587821628851,
1.53206141455895));
#14374=CARTESIAN_POINT('Ctrl Pts',(-19.081438532566,-21.1986129794598,0.187503087496803));
#14375=CARTESIAN_POINT('Ctrl Pts',(-19.0907374657687,-21.2,0.0937256760945715));
#14376=CARTESIAN_POINT('Ctrl Pts',(-19.1,-21.2,4.06896738525122E-13));
#14377=CARTESIAN_POINT('Ctrl Pts',(-16.9,-21.2,-6.93889390390721E-15));
#14378=CARTESIAN_POINT('Ctrl Pts',(-16.8969830453883,-21.2,0.0305279423179293));
#14379=CARTESIAN_POINT('Ctrl Pts',(-16.8939621685952,-21.1998528492313,
0.061061986178125));
#14380=CARTESIAN_POINT('Ctrl Pts',(-16.767248128974,-21.1875162370896,1.34043950276099));
#14381=CARTESIAN_POINT('Ctrl Pts',(-16.6394486076613,-20.929329190971,2.57468702777397));
#14382=CARTESIAN_POINT('Ctrl Pts',(-16.390901029389,-19.9527852055101,4.8667989871523));
#14383=CARTESIAN_POINT('Ctrl Pts',(-16.2661865852166,-19.2459958496645,
5.90361775701928));
#14384=CARTESIAN_POINT('Ctrl Pts',(-16.0164434579476,-17.4760938667978,
7.6434092654843));
#14385=CARTESIAN_POINT('Ctrl Pts',(-15.8942543732133,-16.4310772867914,
8.33076824399953));
#14386=CARTESIAN_POINT('Ctrl Pts',(-15.6437167913769,-14.1377024264444,
9.26493007649789));
#14387=CARTESIAN_POINT('Ctrl Pts',(-15.5228012264078,-12.9114457325454,
9.50334490259744));
#14388=CARTESIAN_POINT('Ctrl Pts',(-15.2718422511462,-10.4357116660551,
9.49658163777807));
#14389=CARTESIAN_POINT('Ctrl Pts',(-15.1508875962576,-9.20987735813003,
9.25110322734293));
#14390=CARTESIAN_POINT('Ctrl Pts',(-14.8998967426513,-6.91855760852222,
8.30236799838261));
#14391=CARTESIAN_POINT('Ctrl Pts',(-14.7776129198827,-5.87549075136833,
7.60702303698604));
#14392=CARTESIAN_POINT('Ctrl Pts',(-14.5269765839982,-4.1122003669309,5.85068851113439));
#14393=CARTESIAN_POINT('Ctrl Pts',(-14.402176887142,-3.41051525358195,4.80513228098767));
#14394=CARTESIAN_POINT('Ctrl Pts',(-14.152310008838,-2.44844277306473,2.49636756975496));
#14395=CARTESIAN_POINT('Ctrl Pts',(-14.0239657950969,-2.19999999999999,
1.25438434751193));
#14396=CARTESIAN_POINT('Ctrl Pts',(-13.7760812749615,-2.20000000000001,
-1.25390805528599));
#14397=CARTESIAN_POINT('Ctrl Pts',(-13.6477361899215,-2.44826489212498,
-2.49594069418698));
#14398=CARTESIAN_POINT('Ctrl Pts',(-13.397823112858,-3.41051525358197,-4.80513228098764));
#14399=CARTESIAN_POINT('Ctrl Pts',(-13.2730234160018,-4.11220036693088,
-5.85068851113436));
#14400=CARTESIAN_POINT('Ctrl Pts',(-13.0223870801173,-5.87549075136848,
-7.60702303698617));
#14401=CARTESIAN_POINT('Ctrl Pts',(-12.9001032573487,-6.9185576085226,-8.30236799838268));
#14402=CARTESIAN_POINT('Ctrl Pts',(-12.6491124037424,-9.20987735813013,
-9.25110322734288));
#14403=CARTESIAN_POINT('Ctrl Pts',(-12.5281577488538,-10.4357116660553,
-9.49658163777797));
#14404=CARTESIAN_POINT('Ctrl Pts',(-12.2771987735922,-12.9114457325455,
-9.50334490259733));
#14405=CARTESIAN_POINT('Ctrl Pts',(-12.156283208623,-14.1377024264445,-9.26493007649772));
#14406=CARTESIAN_POINT('Ctrl Pts',(-11.9057456267867,-16.4310772867914,
-8.33076824399935));
#14407=CARTESIAN_POINT('Ctrl Pts',(-11.7835565420524,-17.4760938667978,
-7.64340926548411));
#14408=CARTESIAN_POINT('Ctrl Pts',(-11.5338134147834,-19.2459958496646,
-5.90361775701905));
#14409=CARTESIAN_POINT('Ctrl Pts',(-11.409098970611,-19.9527852055101,-4.86679898715208));
#14410=CARTESIAN_POINT('Ctrl Pts',(-11.1605513923387,-20.9293291909709,
-2.57468702777379));
#14411=CARTESIAN_POINT('Ctrl Pts',(-11.032751871026,-21.1875162370895,-1.34043950276079));
#14412=CARTESIAN_POINT('Ctrl Pts',(-10.9060378314048,-21.1998528492312,
-0.0610619861779927));
#14413=CARTESIAN_POINT('Ctrl Pts',(-10.9030169546117,-21.2,-0.03052794231788));
#14414=CARTESIAN_POINT('Ctrl Pts',(-10.9,-21.2,-2.0081840286763E-14));
#14415=CARTESIAN_POINT('Origin',(78.0000000000001,-11.7,-3.46944695195361E-15));
#14416=CARTESIAN_POINT('',(-4.90000000000003,-21.2,-1.98093323684911E-13));
#14417=CARTESIAN_POINT('',(-7.1,-21.2,-4.25932099866582E-15));
#14418=CARTESIAN_POINT('',(78.0000000000001,-21.2,-4.6328614111436E-15));
#14419=CARTESIAN_POINT('Ctrl Pts',(-7.1,-21.2,-1.04083408558609E-14));
#14420=CARTESIAN_POINT('Ctrl Pts',(-7.10301695461173,-21.2,-0.0305279423178875));
#14421=CARTESIAN_POINT('Ctrl Pts',(-7.10603783140479,-21.1998528492312,
-0.0610619861780148));
#14422=CARTESIAN_POINT('Ctrl Pts',(-7.23275187102597,-21.1875162370895,
-1.34043950276082));
#14423=CARTESIAN_POINT('Ctrl Pts',(-7.36055139233868,-20.9293291909709,
-2.57468702777381));
#14424=CARTESIAN_POINT('Ctrl Pts',(-7.60909897061095,-19.9527852055101,
-4.86679898715213));
#14425=CARTESIAN_POINT('Ctrl Pts',(-7.73381341478335,-19.2459958496646,
-5.90361775701912));
#14426=CARTESIAN_POINT('Ctrl Pts',(-7.98355654205236,-17.4760938667978,
-7.64340926548419));
#14427=CARTESIAN_POINT('Ctrl Pts',(-8.10574562678669,-16.4310772867913,
-8.33076824399942));
#14428=CARTESIAN_POINT('Ctrl Pts',(-8.35628320862303,-14.1377024264445,
-9.26493007649778));
#14429=CARTESIAN_POINT('Ctrl Pts',(-8.47719877359217,-12.9114457325455,
-9.50334490259736));
#14430=CARTESIAN_POINT('Ctrl Pts',(-8.72815774885374,-10.4357116660555,
-9.49658163777799));
#14431=CARTESIAN_POINT('Ctrl Pts',(-8.84911240374241,-9.2098773581302,-9.25110322734298));
#14432=CARTESIAN_POINT('Ctrl Pts',(-9.10010325734868,-6.91855760852233,
-8.30236799838263));
#14433=CARTESIAN_POINT('Ctrl Pts',(-9.22238708011727,-5.87549075136838,
-7.60702303698608));
#14434=CARTESIAN_POINT('Ctrl Pts',(-9.47302341600179,-4.1122003669308,-5.85068851113429));
#14435=CARTESIAN_POINT('Ctrl Pts',(-9.59782311285803,-3.41051525358196,
-4.80513228098758));
#14436=CARTESIAN_POINT('Ctrl Pts',(-9.84773618992147,-2.44826489212505,
-2.4959406941871));
#14437=CARTESIAN_POINT('Ctrl Pts',(-9.97608127496146,-2.2,-1.25390805528605));
#14438=CARTESIAN_POINT('Ctrl Pts',(-10.2239657950969,-2.19999999999999,
1.25438434751194));
#14439=CARTESIAN_POINT('Ctrl Pts',(-10.352310008838,-2.44844277306475,2.49636756975497));
#14440=CARTESIAN_POINT('Ctrl Pts',(-10.602176887142,-3.41051525358195,4.80513228098765));
#14441=CARTESIAN_POINT('Ctrl Pts',(-10.7269765839982,-4.11220036693091,
5.85068851113438));
#14442=CARTESIAN_POINT('Ctrl Pts',(-10.9776129198827,-5.87549075136841,
7.60702303698611));
#14443=CARTESIAN_POINT('Ctrl Pts',(-11.0998967426514,-6.91855760852248,
8.30236799838264));
#14444=CARTESIAN_POINT('Ctrl Pts',(-11.3508875962576,-9.20987735813005,
9.25110322734288));
#14445=CARTESIAN_POINT('Ctrl Pts',(-11.4718422511462,-10.4357116660552,
9.496581637778));
#14446=CARTESIAN_POINT('Ctrl Pts',(-11.7228012264078,-12.9114457325453,
9.50334490259737));
#14447=CARTESIAN_POINT('Ctrl Pts',(-11.843716791377,-14.1377024264444,9.26493007649785));
#14448=CARTESIAN_POINT('Ctrl Pts',(-12.0942543732133,-16.4310772867913,
8.33076824399947));
#14449=CARTESIAN_POINT('Ctrl Pts',(-12.2164434579477,-17.4760938667978,
7.64340926548424));
#14450=CARTESIAN_POINT('Ctrl Pts',(-12.4661865852167,-19.2459958496646,
5.90361775701917));
#14451=CARTESIAN_POINT('Ctrl Pts',(-12.5909010293891,-19.9527852055101,
4.8667989871522));
#14452=CARTESIAN_POINT('Ctrl Pts',(-12.8394486076613,-20.929329190971,2.57468702777389));
#14453=CARTESIAN_POINT('Ctrl Pts',(-12.9672481289741,-21.1875162370896,
1.3404395027609));
#14454=CARTESIAN_POINT('Ctrl Pts',(-13.0939621685952,-21.1998528492313,
0.0610619861780588));
#14455=CARTESIAN_POINT('Ctrl Pts',(-13.0969830453883,-21.2,0.0305279423179154));
#14456=CARTESIAN_POINT('Ctrl Pts',(-13.1,-21.2,1.94289029309403E-14));
#14457=CARTESIAN_POINT('Ctrl Pts',(-10.9,-21.2,-2.05391259555654E-14));
#14458=CARTESIAN_POINT('Ctrl Pts',(-10.7792854883044,-21.2,1.22148528043648));
#14459=CARTESIAN_POINT('Ctrl Pts',(-10.6543248572149,-20.9644157250573,
2.43216559502755));
#14460=CARTESIAN_POINT('Ctrl Pts',(-10.407311325678,-20.0379796864884,4.72019166334933));
#14461=CARTESIAN_POINT('Ctrl Pts',(-10.2830519498147,-19.3476995003352,
5.77191772591653));
#14462=CARTESIAN_POINT('Ctrl Pts',(-10.0323229281731,-17.6042062462672,
7.54520943878794));
#14463=CARTESIAN_POINT('Ctrl Pts',(-9.91037350082199,-16.5692015069558,
8.25108999017974));
#14464=CARTESIAN_POINT('Ctrl Pts',(-9.65935921798872,-14.2891812567473,
9.22382157527658));
#14465=CARTESIAN_POINT('Ctrl Pts',(-9.53850996698142,-13.0664139465299,
9.48238228915555));
#14466=CARTESIAN_POINT('Ctrl Pts',(-9.28759889551594,-10.5911524555268,
9.51587183654892));
#14467=CARTESIAN_POINT('Ctrl Pts',(-9.16654819825313,-9.36229409907269,
9.29067738573355));
#14468=CARTESIAN_POINT('Ctrl Pts',(-8.91612834663441,-7.05840175783258,
8.38103212678943));
#14469=CARTESIAN_POINT('Ctrl Pts',(-8.79356951655812,-6.00563654506221,
7.70457444607819));
#14470=CARTESIAN_POINT('Ctrl Pts',(-8.54400917814636,-4.21629480933569,
5.9825920401691));
#14471=CARTESIAN_POINT('Ctrl Pts',(-8.41870882166752,-3.49816598006753,
4.95240981504442));
#14472=CARTESIAN_POINT('Ctrl Pts',(-8.17042218264078,-2.49719213060864,
2.6685142031841));
#14473=CARTESIAN_POINT('Ctrl Pts',(-8.04247821816479,-2.22627476101526,
1.43571070081269));
#14474=CARTESIAN_POINT('Ctrl Pts',(-7.7942317997949,-2.17734057865542,-1.0650747678811));
#14475=CARTESIAN_POINT('Ctrl Pts',(-7.66729928940652,-2.40024227986408,
-2.30894656775598));
#14476=CARTESIAN_POINT('Ctrl Pts',(-7.41707867178707,-3.31314727879848,
-4.63251285108605));
#14477=CARTESIAN_POINT('Ctrl Pts',(-7.29333380378853,-3.99170948168244,
-5.69050173900314));
#14478=CARTESIAN_POINT('Ctrl Pts',(-7.04252304168434,-5.71485444423936,
-7.48105206828023));
#14479=CARTESIAN_POINT('Ctrl Pts',(-6.92087304401098,-6.74156121041487,
-8.19766790339084));
#14480=CARTESIAN_POINT('Ctrl Pts',(-6.66984812699976,-9.0099170399785,-9.19486269390227));
#14481=CARTESIAN_POINT('Ctrl Pts',(-6.54906175941734,-10.2294916214264,
-9.46676421981235));
#14482=CARTESIAN_POINT('Ctrl Pts',(-6.29821274278055,-12.7041409356655,
-9.52751127093382));
#14483=CARTESIAN_POINT('Ctrl Pts',(-6.17697944446328,-13.9355883064955,
-9.31580037992587));
#14484=CARTESIAN_POINT('Ctrl Pts',(-5.92669221714971,-16.25007296627,-8.4311657392535));
#14485=CARTESIAN_POINT('Ctrl Pts',(-5.80371405667172,-17.3106672228247,
-7.76583202293341));
#14486=CARTESIAN_POINT('Ctrl Pts',(-5.55435168263951,-19.1196837186765,
-6.06203761529504));
#14487=CARTESIAN_POINT('Ctrl Pts',(-5.42841638903915,-19.8492914847693,
-5.03864619904393));
#14488=CARTESIAN_POINT('Ctrl Pts',(-5.18041429727117,-20.8749735642954,
-2.76326935456374));
#14489=CARTESIAN_POINT('Ctrl Pts',(-5.05233723624973,-21.158782162885,-1.53206141455799));
#14490=CARTESIAN_POINT('Ctrl Pts',(-4.91856146743402,-21.1986129794595,
-0.187503087496173));
#14491=CARTESIAN_POINT('Ctrl Pts',(-4.90926253423129,-21.2,-0.0937256760942467));
#14492=CARTESIAN_POINT('Ctrl Pts',(-4.90000000000004,-21.2,-3.91553785958679E-13));
#14493=CARTESIAN_POINT('Origin',(78.0000000000001,-11.7,-3.46944695195361E-15));
#14494=CARTESIAN_POINT('',(1.10000000000044,-21.2,2.23339518513334E-12));
#14495=CARTESIAN_POINT('',(-1.10000000000004,-21.2,-2.02746363044123E-13));
#14496=CARTESIAN_POINT('',(78.0000000000001,-21.2,-4.6328614111436E-15));
#14497=CARTESIAN_POINT('Ctrl Pts',(-1.10000000000004,-21.2,-4.00859864677103E-13));
#14498=CARTESIAN_POINT('Ctrl Pts',(-1.10926253423131,-21.2,-0.0937256760943962));
#14499=CARTESIAN_POINT('Ctrl Pts',(-1.11856146743405,-21.1986129794596,
-0.187503087496459));
#14500=CARTESIAN_POINT('Ctrl Pts',(-1.25233723624978,-21.158782162885,-1.53206141455843));
#14501=CARTESIAN_POINT('Ctrl Pts',(-1.38041429727121,-20.8749735642953,
-2.76326935456418));
#14502=CARTESIAN_POINT('Ctrl Pts',(-1.62841638903919,-19.8492914847691,
-5.03864619904435));
#14503=CARTESIAN_POINT('Ctrl Pts',(-1.75435168263955,-19.1196837186762,
-6.06203761529545));
#14504=CARTESIAN_POINT('Ctrl Pts',(-2.00371405667176,-17.3106672228244,
-7.76583202293368));
#14505=CARTESIAN_POINT('Ctrl Pts',(-2.12669221714973,-16.2500729662697,
-8.43116573925373));
#14506=CARTESIAN_POINT('Ctrl Pts',(-2.37697944446329,-13.9355883064952,
-9.315800379926));
#14507=CARTESIAN_POINT('Ctrl Pts',(-2.49821274278056,-12.7041409356653,
-9.52751127093395));
#14508=CARTESIAN_POINT('Ctrl Pts',(-2.74906175941735,-10.2294916214261,
-9.46676421981238));
#14509=CARTESIAN_POINT('Ctrl Pts',(-2.86984812699978,-9.00991703997814,
-9.19486269390226));
#14510=CARTESIAN_POINT('Ctrl Pts',(-3.12087304401099,-6.74156121041458,
-8.19766790339077));
#14511=CARTESIAN_POINT('Ctrl Pts',(-3.24252304168436,-5.71485444423907,
-7.48105206828013));
#14512=CARTESIAN_POINT('Ctrl Pts',(-3.49333380378854,-3.9917094816822,-5.69050173900298));
#14513=CARTESIAN_POINT('Ctrl Pts',(-3.61707867178709,-3.31314727879827,
-4.63251285108587));
#14514=CARTESIAN_POINT('Ctrl Pts',(-3.86729928940655,-2.40024227986389,
-2.30894656775566));
#14515=CARTESIAN_POINT('Ctrl Pts',(-3.99423179979492,-2.17734057865532,
-1.06507476788081));
#14516=CARTESIAN_POINT('Ctrl Pts',(-4.24247821816481,-2.22627476101522,
1.43571070081288));
#14517=CARTESIAN_POINT('Ctrl Pts',(-4.3704221826408,-2.49719213060861,2.66851420318427));
#14518=CARTESIAN_POINT('Ctrl Pts',(-4.61870882166753,-3.49816598006755,
4.95240981504459));
#14519=CARTESIAN_POINT('Ctrl Pts',(-4.74400917814637,-4.21629480933573,
5.98259204016927));
#14520=CARTESIAN_POINT('Ctrl Pts',(-4.99356951655813,-6.00563654506232,
7.70457444607837));
#14521=CARTESIAN_POINT('Ctrl Pts',(-5.11612834663442,-7.05840175783277,
8.38103212678959));
#14522=CARTESIAN_POINT('Ctrl Pts',(-5.36654819825314,-9.36229409907284,
9.29067738573365));
#14523=CARTESIAN_POINT('Ctrl Pts',(-5.48759889551595,-10.591152455527,9.51587183654897));
#14524=CARTESIAN_POINT('Ctrl Pts',(-5.73850996698142,-13.06641394653,9.48238228915556));
#14525=CARTESIAN_POINT('Ctrl Pts',(-5.85935921798873,-14.2891812567474,
9.22382157527661));
#14526=CARTESIAN_POINT('Ctrl Pts',(-6.11037350082199,-16.5692015069559,
8.25108999017975));
#14527=CARTESIAN_POINT('Ctrl Pts',(-6.23232292817312,-17.6042062462673,
7.54520943878795));
#14528=CARTESIAN_POINT('Ctrl Pts',(-6.48305194981473,-19.3476995003354,
5.77191772591646));
#14529=CARTESIAN_POINT('Ctrl Pts',(-6.60731132567798,-20.0379796864884,
4.72019166334927));
#14530=CARTESIAN_POINT('Ctrl Pts',(-6.85432485721487,-20.9644157250573,
2.43216559502755));
#14531=CARTESIAN_POINT('Ctrl Pts',(-6.97928548830439,-21.2,1.22148528043648));
#14532=CARTESIAN_POINT('Ctrl Pts',(-7.1,-21.2,-9.71445146547012E-15));
#14533=CARTESIAN_POINT('',(-1.9,-2.2,0.));
#14534=CARTESIAN_POINT('Ctrl Pts',(-4.90000000000003,-21.2,-3.92186283448837E-13));
#14535=CARTESIAN_POINT('Ctrl Pts',(-4.78589463992307,-21.2,1.15460863648533));
#14536=CARTESIAN_POINT('Ctrl Pts',(-4.66790884158497,-20.9895203441914,
2.30044202055665));
#14537=CARTESIAN_POINT('Ctrl Pts',(-4.42697349753129,-20.1352887413487,
4.54344435292883));
#14538=CARTESIAN_POINT('Ctrl Pts',(-4.30370702740743,-19.468575729199,5.6076889832996));
#14539=CARTESIAN_POINT('Ctrl Pts',(-4.0528272950289,-17.7660153225651,7.41552521022513));
#14540=CARTESIAN_POINT('Ctrl Pts',(-3.93143494871502,-16.7477137680786,
8.14290619632631));
#14541=CARTESIAN_POINT('Ctrl Pts',(-3.68041314308496,-14.491210884508,9.16464314019071));
#14542=CARTESIAN_POINT('Ctrl Pts',(-3.55964376528457,-13.2749008689796,
9.44993444082394));
#14543=CARTESIAN_POINT('Ctrl Pts',(-3.30887066922413,-10.8010005184188,
9.53803958026867));
#14544=CARTESIAN_POINT('Ctrl Pts',(-3.18740883981607,-9.56702001222297,
9.33986229220452));
#14545=CARTESIAN_POINT('Ctrl Pts',(-2.93726735399162,-7.24203907542668,
8.48033707933681));
#14546=CARTESIAN_POINT('Ctrl Pts',(-2.81382602429882,-6.17366151377793,
7.82617419694249));
#14547=CARTESIAN_POINT('Ctrl Pts',(-2.56467391769076,-4.34505010391411,
6.14065935137722));
#14548=CARTESIAN_POINT('Ctrl Pts',(-2.43806428423111,-3.60400801504371,
5.12410600030631));
#14549=CARTESIAN_POINT('Ctrl Pts',(-2.24634089916518,-2.79107732111404,
3.36964268186199));
#14550=CARTESIAN_POINT('Ctrl Pts',(-2.17675453192557,-2.57052382279359,
2.71585246112379));
#14551=CARTESIAN_POINT('Ctrl Pts',(-2.03735749352367,-2.27462673223717,
1.37285912097279));
#14552=CARTESIAN_POINT('Ctrl Pts',(-1.96794156984213,-2.20000000000001,
0.687486751395415));
#14553=CARTESIAN_POINT('Ctrl Pts',(-1.9,-2.20000000000001,0.));
#14554=CARTESIAN_POINT('Ctrl Pts',(-1.9,-2.20000000000001,-9.71445146547012E-16));
#14555=CARTESIAN_POINT('Ctrl Pts',(-1.82240919606718,-2.20000000000001,
-0.785125363718995));
#14556=CARTESIAN_POINT('Ctrl Pts',(-1.742931224028,-2.29732921818939,-1.56713183388941));
#14557=CARTESIAN_POINT('Ctrl Pts',(-1.58397810910787,-2.68171790682092,
-3.08781145458966));
#14558=CARTESIAN_POINT('Ctrl Pts',(-1.50627788561728,-2.96698552223606,
-3.82077835789411));
#14559=CARTESIAN_POINT('Ctrl Pts',(-1.30309366168197,-3.93400067098277,
-5.61337377836322));
#14560=CARTESIAN_POINT('Ctrl Pts',(-1.17482924813685,-4.74147972021909,
-6.5878620867794));
#14561=CARTESIAN_POINT('Ctrl Pts',(-0.927331863007985,-6.68268234478074,
-8.16270927538555));
#14562=CARTESIAN_POINT('Ctrl Pts',(-0.800278464085321,-7.79598298912007,
-8.75006417475044));
#14563=CARTESIAN_POINT('Ctrl Pts',(-0.551264801242581,-10.1808762870929,
-9.45953708808233));
#14564=CARTESIAN_POINT('Ctrl Pts',(-0.427510001032243,-11.4286112335544,
-9.57690646451572));
#14565=CARTESIAN_POINT('Ctrl Pts',(-0.177466838670091,-13.8953107190287,
-9.32543555556563));
#14566=CARTESIAN_POINT('Ctrl Pts',(-0.0558377561646816,-15.090781291844,
-8.96021822335387));
#14567=CARTESIAN_POINT('Ctrl Pts',(0.194880480566995,-17.273490661377,-7.79214963085964));
#14568=CARTESIAN_POINT('Ctrl Pts',(0.315662999058585,-18.2400206930619,
-7.00067537881007));
#14569=CARTESIAN_POINT('Ctrl Pts',(0.566675728348146,-19.8162347312299,
-5.09040313956777));
#14570=CARTESIAN_POINT('Ctrl Pts',(0.687928012700195,-20.4103423716323,
-3.98943736487644));
#14571=CARTESIAN_POINT('Ctrl Pts',(0.909485604799865,-21.0576446211017,
-1.89528423874928));
#14572=CARTESIAN_POINT('Ctrl Pts',(1.00615236670273,-21.2,-0.949624871658705));
#14573=CARTESIAN_POINT('Ctrl Pts',(1.10000000000044,-21.2,4.47988868224058E-12));
#14574=CARTESIAN_POINT('Origin',(78.0000000000001,-11.7,-3.46944695195361E-15));
#14575=CARTESIAN_POINT('',(7.10000000000035,-21.2,1.74965019662244E-12));
#14576=CARTESIAN_POINT('',(4.90000000000003,-21.2,1.91358318085311E-13));
#14577=CARTESIAN_POINT('',(78.0000000000001,-21.2,-4.6328614111436E-15));
#14578=CARTESIAN_POINT('',(1.9,-2.19999999999999,0.));
#14579=CARTESIAN_POINT('Ctrl Pts',(4.90000000000004,-21.2,3.87190279838023E-13));
#14580=CARTESIAN_POINT('Ctrl Pts',(4.78589463992312,-21.2,-1.15460863648501));
#14581=CARTESIAN_POINT('Ctrl Pts',(4.66790884158501,-20.9895203441916,-2.30044202055602));
#14582=CARTESIAN_POINT('Ctrl Pts',(4.42697349753135,-20.1352887413493,-4.54344435292803));
#14583=CARTESIAN_POINT('Ctrl Pts',(4.30370702740749,-19.4685757291996,-5.60768898329891));
#14584=CARTESIAN_POINT('Ctrl Pts',(4.05282729502898,-17.7660153225659,-7.41552521022458));
#14585=CARTESIAN_POINT('Ctrl Pts',(3.9314349487151,-16.7477137680793,-8.14290619632586));
#14586=CARTESIAN_POINT('Ctrl Pts',(3.68041314308507,-14.4912108845091,-9.16464314019039));
#14587=CARTESIAN_POINT('Ctrl Pts',(3.55964376528467,-13.2749008689808,-9.44993444082381));
#14588=CARTESIAN_POINT('Ctrl Pts',(3.30887066922423,-10.8010005184199,-9.53803958026883));
#14589=CARTESIAN_POINT('Ctrl Pts',(3.18740883981617,-9.56702001222408,-9.33986229220482));
#14590=CARTESIAN_POINT('Ctrl Pts',(2.93726735399172,-7.24203907542763,-8.48033707933737));
#14591=CARTESIAN_POINT('Ctrl Pts',(2.81382602429894,-6.17366151377884,-7.82617419694316));
#14592=CARTESIAN_POINT('Ctrl Pts',(2.56467391769087,-4.34505010391488,-6.14065935137818));
#14593=CARTESIAN_POINT('Ctrl Pts',(2.43806428423122,-3.60400801504429,-5.12410600030733));
#14594=CARTESIAN_POINT('Ctrl Pts',(2.24634089916526,-2.79107732111432,-3.36964268186288));
#14595=CARTESIAN_POINT('Ctrl Pts',(2.17675453192563,-2.57052382279375,-2.71585246112451));
#14596=CARTESIAN_POINT('Ctrl Pts',(2.03735749352367,-2.2746267322371,-1.37285912097289));
#14597=CARTESIAN_POINT('Ctrl Pts',(1.96794156984213,-2.20000000000001,-0.687486751395457));
#14598=CARTESIAN_POINT('Ctrl Pts',(1.9,-2.20000000000001,4.16333634234434E-16));
#14599=CARTESIAN_POINT('Ctrl Pts',(1.9,-2.20000000000001,2.77555756156289E-16));
#14600=CARTESIAN_POINT('Ctrl Pts',(1.8320584301579,-2.20000000000001,0.687486751395224));
#14601=CARTESIAN_POINT('Ctrl Pts',(1.76264250647639,-2.27462673223699,1.37285912097244));
#14602=CARTESIAN_POINT('Ctrl Pts',(1.62324546807441,-2.57052382279363,2.7158524611242));
#14603=CARTESIAN_POINT('Ctrl Pts',(1.55365910083479,-2.79107732111415,3.36964268186248));
#14604=CARTESIAN_POINT('Ctrl Pts',(1.36193571576884,-3.60400801504399,5.1241060003069));
#14605=CARTESIAN_POINT('Ctrl Pts',(1.23532608230919,-4.34505010391456,6.14065935137781));
#14606=CARTESIAN_POINT('Ctrl Pts',(0.986173975701136,-6.17366151377839,
7.82617419694286));
#14607=CARTESIAN_POINT('Ctrl Pts',(0.862732646008349,-7.24203907542715,
8.48033707933712));
#14608=CARTESIAN_POINT('Ctrl Pts',(0.612591160183894,-9.56702001222349,
9.33986229220469));
#14609=CARTESIAN_POINT('Ctrl Pts',(0.491129330775837,-10.8010005184193,
9.5380395802688));
#14610=CARTESIAN_POINT('Ctrl Pts',(0.240356234715391,-13.2749008689802,
9.44993444082392));
#14611=CARTESIAN_POINT('Ctrl Pts',(0.119586856914992,-14.4912108845086,
9.16464314019056));
#14612=CARTESIAN_POINT('Ctrl Pts',(-0.131434948715058,-16.7477137680791,
8.14290619632607));
#14613=CARTESIAN_POINT('Ctrl Pts',(-0.252827295028933,-17.7660153225655,
7.41552521022482));
#14614=CARTESIAN_POINT('Ctrl Pts',(-0.503707027407458,-19.4685757291994,
5.60768898329921));
#14615=CARTESIAN_POINT('Ctrl Pts',(-0.626973497531317,-20.135288741349,
4.54344435292839));
#14616=CARTESIAN_POINT('Ctrl Pts',(-0.867908841584979,-20.9895203441915,
2.30044202055641));
#14617=CARTESIAN_POINT('Ctrl Pts',(-0.985894639923092,-21.2,1.15460863648521));
#14618=CARTESIAN_POINT('Ctrl Pts',(-1.10000000000004,-21.2,-3.99957844621213E-13));
#14619=CARTESIAN_POINT('Ctrl Pts',(1.10000000000044,-21.2,4.47669679104479E-12));
#14620=CARTESIAN_POINT('Ctrl Pts',(1.12861197762933,-21.2,0.289518708458957));
#14621=CARTESIAN_POINT('Ctrl Pts',(1.15755311853428,-21.1867657550865,0.579347522267127));
#14622=CARTESIAN_POINT('Ctrl Pts',(1.31226798453121,-21.0459766280402,2.11274118535634));
#14623=CARTESIAN_POINT('Ctrl Pts',(1.43812594008345,-20.687408477367,3.32214218001096));
#14624=CARTESIAN_POINT('Ctrl Pts',(1.68717348681367,-19.5218084280711,5.5350716129601));
#14625=CARTESIAN_POINT('Ctrl Pts',(1.81532810695294,-18.7250004034997,6.51668441409436));
#14626=CARTESIAN_POINT('Ctrl Pts',(2.06313890932384,-16.8019149156045,8.10993421382391));
#14627=CARTESIAN_POINT('Ctrl Pts',(2.18949911840483,-15.6958499037577,8.70833285820448));
#14628=CARTESIAN_POINT('Ctrl Pts',(2.43872900929925,-13.320528711054,9.44259877042744));
#14629=CARTESIAN_POINT('Ctrl Pts',(2.5619970700894,-12.0749025039173,9.57331164819956));
#14630=CARTESIAN_POINT('Ctrl Pts',(2.81219300304181,-9.60669592209691,9.34882097078356));
#14631=CARTESIAN_POINT('Ctrl Pts',(2.93356650916228,-8.40761994419821,8.99679824400882));
#14632=CARTESIAN_POINT('Ctrl Pts',(3.18436883977102,-6.21236435328532,7.85287012939994));
#14633=CARTESIAN_POINT('Ctrl Pts',(3.3051389283296,-5.23710293161833,7.07196332583943));
#14634=CARTESIAN_POINT('Ctrl Pts',(3.55616351811101,-3.6396095638801,5.17851113080937));
#14635=CARTESIAN_POINT('Ctrl Pts',(3.67764453489987,-3.0332911184828,4.0835346992797));
#14636=CARTESIAN_POINT('Ctrl Pts',(3.92850071102958,-2.27424266566553,1.71842057764594));
#14637=CARTESIAN_POINT('Ctrl Pts',(4.05193666142919,-2.13043722405992,0.470465773785534));
#14638=CARTESIAN_POINT('Ctrl Pts',(4.30224631097138,-2.33254511812152,-2.01623620603559));
#14639=CARTESIAN_POINT('Ctrl Pts',(4.42874911942666,-2.67908579453452,-3.23054604201975));
#14640=CARTESIAN_POINT('Ctrl Pts',(4.67731276154541,-3.82242011052979,-5.45512593035675));
#14641=CARTESIAN_POINT('Ctrl Pts',(4.80534284562397,-4.60834831586048,-6.44384371054323));
#14642=CARTESIAN_POINT('Ctrl Pts',(5.05345105369771,-6.51294888414738,-8.05558738602805));
#14643=CARTESIAN_POINT('Ctrl Pts',(5.17914998170505,-7.61164297709098,-8.66512040772011));
#14644=CARTESIAN_POINT('Ctrl Pts',(5.42858604607204,-9.97718208881188,-9.42438672970812));
#14645=CARTESIAN_POINT('Ctrl Pts',(5.5514060490949,-11.2206160705921,-9.56855818217814));
#14646=CARTESIAN_POINT('Ctrl Pts',(5.80174320770436,-13.6902158568989,-9.37127791725014));
#14647=CARTESIAN_POINT('Ctrl Pts',(5.92290454188791,-14.8928618977337,-9.03256486454203));
#14648=CARTESIAN_POINT('Ctrl Pts',(6.17377777989577,-17.1006241722849,-7.91299494415882));
#14649=CARTESIAN_POINT('Ctrl Pts',(6.2945818874263,-18.0846226647122,-7.14274957259232));
#14650=CARTESIAN_POINT('Ctrl Pts',(6.54560447338455,-19.7034081654102,-5.2663025710902));
#14651=CARTESIAN_POINT('Ctrl Pts',(6.66735898898658,-20.3219530488362,-4.17739679312542));
#14652=CARTESIAN_POINT('Ctrl Pts',(6.89553917980856,-21.0362589525294,-2.03152410141216));
#14653=CARTESIAN_POINT('Ctrl Pts',(6.99935185262614,-21.2,-1.01843787290684));
#14654=CARTESIAN_POINT('Ctrl Pts',(7.10000000000035,-21.2,3.51135787113321E-12));
#14655=CARTESIAN_POINT('Origin',(78.0000000000001,-11.7,-3.46944695195361E-15));
#14656=CARTESIAN_POINT('',(13.1000000000002,-21.2,7.83235748155766E-13));
#14657=CARTESIAN_POINT('',(10.9,-21.2,7.85595533902485E-16));
#14658=CARTESIAN_POINT('',(78.0000000000001,-21.2,-4.6328614111436E-15));
#14659=CARTESIAN_POINT('Ctrl Pts',(10.9,-21.2,7.7715611723761E-15));
#14660=CARTESIAN_POINT('Ctrl Pts',(10.7792854883044,-21.2,-1.22148528043641));
#14661=CARTESIAN_POINT('Ctrl Pts',(10.6543248572149,-20.9644157250575,-2.4321655950274));
#14662=CARTESIAN_POINT('Ctrl Pts',(10.407311325678,-20.0379796864886,-4.72019166334919));
#14663=CARTESIAN_POINT('Ctrl Pts',(10.2830519498147,-19.3476995003354,-5.77191772591644));
#14664=CARTESIAN_POINT('Ctrl Pts',(10.0323229281731,-17.6042062462675,-7.54520943878787));
#14665=CARTESIAN_POINT('Ctrl Pts',(9.91037350082199,-16.569201506956,-8.25108999017969));
#14666=CARTESIAN_POINT('Ctrl Pts',(9.65935921798875,-14.2891812567478,-9.22382157527654));
#14667=CARTESIAN_POINT('Ctrl Pts',(9.53850996698144,-13.0664139465303,-9.48238228915556));
#14668=CARTESIAN_POINT('Ctrl Pts',(9.28759889551597,-10.5911524555272,-9.51587183654906));
#14669=CARTESIAN_POINT('Ctrl Pts',(9.16654819825315,-9.36229409907313,-9.29067738573375));
#14670=CARTESIAN_POINT('Ctrl Pts',(8.91612834663444,-7.05840175783301,-8.38103212678977));
#14671=CARTESIAN_POINT('Ctrl Pts',(8.79356951655815,-6.00563654506256,-7.70457444607858));
#14672=CARTESIAN_POINT('Ctrl Pts',(8.54400917814639,-4.21629480933593,-5.98259204016955));
#14673=CARTESIAN_POINT('Ctrl Pts',(8.41870882166755,-3.49816598006771,-4.9524098150449));
#14674=CARTESIAN_POINT('Ctrl Pts',(8.17042218264081,-2.49719213060868,-2.66851420318459));
#14675=CARTESIAN_POINT('Ctrl Pts',(8.04247821816483,-2.22627476101527,-1.43571070081323));
#14676=CARTESIAN_POINT('Ctrl Pts',(7.79423179979495,-2.17734057865527,1.06507476788044));
#14677=CARTESIAN_POINT('Ctrl Pts',(7.66729928940657,-2.4002422798638,2.3089465677553));
#14678=CARTESIAN_POINT('Ctrl Pts',(7.41707867178712,-3.31314727879806,4.63251285108547));
#14679=CARTESIAN_POINT('Ctrl Pts',(7.29333380378858,-3.99170948168188,5.69050173900259));
#14680=CARTESIAN_POINT('Ctrl Pts',(7.04252304168439,-5.71485444423867,7.48105206827982));
#14681=CARTESIAN_POINT('Ctrl Pts',(6.92087304401103,-6.74156121041404,8.19766790339052));
#14682=CARTESIAN_POINT('Ctrl Pts',(6.6698481269998,-9.0099170399777,9.19486269390218));
#14683=CARTESIAN_POINT('Ctrl Pts',(6.54906175941738,-10.2294916214256,9.46676421981236));
#14684=CARTESIAN_POINT('Ctrl Pts',(6.29821274278059,-12.7041409356648,9.52751127093405));
#14685=CARTESIAN_POINT('Ctrl Pts',(6.17697944446333,-13.9355883064947,9.31580037992616));
#14686=CARTESIAN_POINT('Ctrl Pts',(5.92669221714976,-16.2500729662693,8.431165739254));
#14687=CARTESIAN_POINT('Ctrl Pts',(5.80371405667179,-17.3106672228241,7.765832022934));
#14688=CARTESIAN_POINT('Ctrl Pts',(5.55435168263957,-19.1196837186759,6.06203761529587));
#14689=CARTESIAN_POINT('Ctrl Pts',(5.42841638903921,-19.8492914847689,5.03864619904479));
#14690=CARTESIAN_POINT('Ctrl Pts',(5.18041429727123,-20.8749735642952,2.76326935456466));
#14691=CARTESIAN_POINT('Ctrl Pts',(5.0523372362498,-21.158782162885,1.53206141455891));
#14692=CARTESIAN_POINT('Ctrl Pts',(4.91856146743405,-21.1986129794596,0.187503087496786));
#14693=CARTESIAN_POINT('Ctrl Pts',(4.90926253423132,-21.2,0.0937256760945501));
#14694=CARTESIAN_POINT('Ctrl Pts',(4.90000000000004,-21.2,3.87349497581765E-13));
#14695=CARTESIAN_POINT('Ctrl Pts',(7.10000000000035,-21.2,3.5166661249697E-12));
#14696=CARTESIAN_POINT('Ctrl Pts',(7.12207987122531,-21.2,0.223421669166213));
#14697=CARTESIAN_POINT('Ctrl Pts',(7.14435953967788,-21.1921185564034,0.44706615725391));
#14698=CARTESIAN_POINT('Ctrl Pts',(7.29223738335333,-21.0879231886111,1.91962968643776));
#14699=CARTESIAN_POINT('Ctrl Pts',(7.4194215259546,-20.7534347853916,3.13878541973641));
#14700=CARTESIAN_POINT('Ctrl Pts',(7.66748388707429,-19.6323975705467,5.37482152444833));
#14701=CARTESIAN_POINT('Ctrl Pts',(7.79537640986638,-18.8573834318446,6.3705072436837));
#14702=CARTESIAN_POINT('Ctrl Pts',(8.04376099233663,-16.971339193686,8.00053637136689));
#14703=CARTESIAN_POINT('Ctrl Pts',(8.16884187858872,-15.8800332301411,8.62111552010978));
#14704=CARTESIAN_POINT('Ctrl Pts',(8.41847066603455,-13.5243301865345,9.40518853940912));
#14705=CARTESIAN_POINT('Ctrl Pts',(8.54088889269013,-12.2831366735295,9.56271760385075));
#14706=CARTESIAN_POINT('Ctrl Pts',(8.79149441040546,-9.81088949960649,9.39234590031904));
#14707=CARTESIAN_POINT('Ctrl Pts',(8.91262867718373,-8.60345185493481,9.06620679395304));
#14708=CARTESIAN_POINT('Ctrl Pts',(9.16362762048596,-6.38328003924247,7.96954742471251));
#14709=CARTESIAN_POINT('Ctrl Pts',(9.28443993174331,-5.39150745569497,7.21000831202632));
#14710=CARTESIAN_POINT('Ctrl Pts',(9.53510054053434,-3.75443704287751,5.3527104438323));
#14711=CARTESIAN_POINT('Ctrl Pts',(9.65690697436105,-3.12503593325824,4.27243364780206));
#14712=CARTESIAN_POINT('Ctrl Pts',(9.90685108889982,-2.31520599857457,1.92813903140674));
#14713=CARTESIAN_POINT('Ctrl Pts',(10.0309222657915,-2.14380040857977,0.686156174599459));
#14714=CARTESIAN_POINT('Ctrl Pts',(10.2797987797144,-2.28882098605427,-1.7990740085523));
#14715=CARTESIAN_POINT('Ctrl Pts',(10.407291499593,-2.60619987947592,-3.01791987958328));
#14716=CARTESIAN_POINT('Ctrl Pts',(10.6545894668201,-3.69624114641017,-5.26902935946357));
#14717=CARTESIAN_POINT('Ctrl Pts',(10.7829140402373,-4.46092664668805,-6.27840347743013));
#14718=CARTESIAN_POINT('Ctrl Pts',(11.0326896878941,-6.33288154406691,-7.93722084228424));
#14719=CARTESIAN_POINT('Ctrl Pts',(11.1576048875106,-7.42028041952419,-8.57262399701104));
#14720=CARTESIAN_POINT('Ctrl Pts',(11.4082206192069,-9.77313248509324,-9.38505701203718));
#14721=CARTESIAN_POINT('Ctrl Pts',(11.5305782041576,-11.0151474070822,-9.55630141627986));
#14722=CARTESIAN_POINT('Ctrl Pts',(11.7815626432234,-13.491132676413,-9.41146479449907));
#14723=CARTESIAN_POINT('Ctrl Pts',(11.9025443344209,-14.7014737928496,-9.09806778344008));
#14724=CARTESIAN_POINT('Ctrl Pts',(12.1535115728152,-16.9326549830229,-8.02499048160666));
#14725=CARTESIAN_POINT('Ctrl Pts',(12.2744047432598,-17.9323602347771,-7.27591812466932));
#14726=CARTESIAN_POINT('Ctrl Pts',(12.5249650266106,-19.58914911386,-5.4356111079513));
#14727=CARTESIAN_POINT('Ctrl Pts',(12.6470831688779,-20.2300252432785,-4.36158171888695));
#14728=CARTESIAN_POINT('Ctrl Pts',(12.8814900909201,-21.0132140553034,-2.1684240907917));
#14729=CARTESIAN_POINT('Ctrl Pts',(12.992505504308,-21.2,-1.08771466140479));
#14730=CARTESIAN_POINT('Ctrl Pts',(13.1000000000002,-21.2,1.5656920204776E-12));
#14731=CARTESIAN_POINT('Origin',(78.0000000000001,-11.7,-3.46944695195361E-15));
#14732=CARTESIAN_POINT('',(28.,-21.2,-4.6328614111436E-15));
#14733=CARTESIAN_POINT('Origin',(28.,-11.7,-6.93889390390723E-15));
#14734=CARTESIAN_POINT('',(22.9,-21.2,-1.91609456404162E-13));
#14735=CARTESIAN_POINT('',(78.0000000000001,-21.2,-4.6328614111436E-15));
#14736=CARTESIAN_POINT('',(16.9,-21.2,-2.31643070557181E-15));
#14737=CARTESIAN_POINT('Ctrl Pts',(22.9,-21.2,-3.7858605139718E-13));
#14738=CARTESIAN_POINT('Ctrl Pts',(22.8907374657687,-21.2,-0.0937256760943193));
#14739=CARTESIAN_POINT('Ctrl Pts',(22.881438532566,-21.1986129794595,-0.187503087496334));
#14740=CARTESIAN_POINT('Ctrl Pts',(22.7476627637503,-21.158782162885,-1.53206141455819));
#14741=CARTESIAN_POINT('Ctrl Pts',(22.6195857027288,-20.8749735642953,-2.76326935456397));
#14742=CARTESIAN_POINT('Ctrl Pts',(22.3715836109608,-19.8492914847691,-5.03864619904417));
#14743=CARTESIAN_POINT('Ctrl Pts',(22.2456483173605,-19.1196837186763,-6.06203761529527));
#14744=CARTESIAN_POINT('Ctrl Pts',(21.9962859433283,-17.3106672228245,-7.76583202293353));
#14745=CARTESIAN_POINT('Ctrl Pts',(21.8733077828503,-16.2500729662698,-8.43116573925361));
#14746=CARTESIAN_POINT('Ctrl Pts',(21.6230205555367,-13.9355883064952,-9.31580037992593));
#14747=CARTESIAN_POINT('Ctrl Pts',(21.5017872572195,-12.7041409356653,-9.52751127093387));
#14748=CARTESIAN_POINT('Ctrl Pts',(21.2509382405827,-10.2294916214262,-9.46676421981232));
#14749=CARTESIAN_POINT('Ctrl Pts',(21.1301518730002,-9.00991703997824,-9.19486269390221));
#14750=CARTESIAN_POINT('Ctrl Pts',(20.879126955989,-6.74156121041469,-8.19766790339075));
#14751=CARTESIAN_POINT('Ctrl Pts',(20.7574769583157,-5.71485444423917,-7.48105206828012));
#14752=CARTESIAN_POINT('Ctrl Pts',(20.5066661962115,-3.9917094816822,-5.69050173900289));
#14753=CARTESIAN_POINT('Ctrl Pts',(20.3829213282129,-3.31314727879835,-4.63251285108579));
#14754=CARTESIAN_POINT('Ctrl Pts',(20.1327007105935,-2.40024227986406,-2.30894656775584));
#14755=CARTESIAN_POINT('Ctrl Pts',(20.0057682002051,-2.17734057865537,-1.06507476788092));
#14756=CARTESIAN_POINT('Ctrl Pts',(19.7575217818352,-2.22627476101527,1.43571070081289));
#14757=CARTESIAN_POINT('Ctrl Pts',(19.6295778173592,-2.49719213060867,2.66851420318429));
#14758=CARTESIAN_POINT('Ctrl Pts',(19.3812911783325,-3.49816598006761,4.9524098150446));
#14759=CARTESIAN_POINT('Ctrl Pts',(19.2559908218536,-4.21629480933581,5.98259204016927));
#14760=CARTESIAN_POINT('Ctrl Pts',(19.0064304834419,-6.00563654506237,7.70457444607833));
#14761=CARTESIAN_POINT('Ctrl Pts',(18.8838716533656,-7.05840175783278,8.38103212678955));
#14762=CARTESIAN_POINT('Ctrl Pts',(18.6334518017469,-9.36229409907291,9.29067738573362));
#14763=CARTESIAN_POINT('Ctrl Pts',(18.512401104484,-10.591152455527,9.51587183654894));
#14764=CARTESIAN_POINT('Ctrl Pts',(18.2614900330186,-13.06641394653,9.48238228915551));
#14765=CARTESIAN_POINT('Ctrl Pts',(18.1406407820113,-14.2891812567475,9.22382157527653));
#14766=CARTESIAN_POINT('Ctrl Pts',(17.889626499178,-16.5692015069559,8.25108999017968));
#14767=CARTESIAN_POINT('Ctrl Pts',(17.7676770718269,-17.6042062462674,7.54520943878787));
#14768=CARTESIAN_POINT('Ctrl Pts',(17.5169480501853,-19.3476995003353,5.77191772591642));
#14769=CARTESIAN_POINT('Ctrl Pts',(17.392688674322,-20.0379796864885,4.72019166334919));
#14770=CARTESIAN_POINT('Ctrl Pts',(17.1456751427851,-20.9644157250573,2.4321655950276));
#14771=CARTESIAN_POINT('Ctrl Pts',(17.0207145116956,-21.2,1.22148528043652));
#14772=CARTESIAN_POINT('Ctrl Pts',(16.9,-21.2,8.32667268468867E-16));
#14773=CARTESIAN_POINT('',(19.1,-21.2,1.55474016669278E-13));
#14774=CARTESIAN_POINT('',(78.0000000000001,-21.2,-4.6328614111436E-15));
#14775=CARTESIAN_POINT('',(22.1,-2.2,0.));
#14776=CARTESIAN_POINT('Ctrl Pts',(19.1,-21.2,3.155808947497E-13));
#14777=CARTESIAN_POINT('Ctrl Pts',(19.1085990463697,-21.2,0.0870119790806313));
#14778=CARTESIAN_POINT('Ctrl Pts',(19.117229491272,-21.1988045700926,0.174068824370104));
#14779=CARTESIAN_POINT('Ctrl Pts',(19.250254599823,-21.1620196858175,1.51172658899612));
#14780=CARTESIAN_POINT('Ctrl Pts',(19.3783048394584,-20.8809326818491,2.74328431513305));
#14781=CARTESIAN_POINT('Ctrl Pts',(19.6269445678301,-19.8580958285676,5.02576267739737));
#14782=CARTESIAN_POINT('Ctrl Pts',(19.7533450987224,-19.1265285069368,6.05479514661026));
#14783=CARTESIAN_POINT('Ctrl Pts',(20.0036755920597,-17.3113998082999,7.76593089658135));
#14784=CARTESIAN_POINT('Ctrl Pts',(20.1270389541067,-16.2472803988743,8.43325057572791));
#14785=CARTESIAN_POINT('Ctrl Pts',(20.3779053449636,-13.9266113917878,9.31821156840541));
#14786=CARTESIAN_POINT('Ctrl Pts',(20.499348010147,-12.6929414155417,9.52894055092275));
#14787=CARTESIAN_POINT('Ctrl Pts',(20.7503716367565,-10.2165695573798,9.46472746246329));
#14788=CARTESIAN_POINT('Ctrl Pts',(20.8711406833289,-8.99752494041226,9.191206657545));
#14789=CARTESIAN_POINT('Ctrl Pts',(21.1219308163566,-6.73272231199642,8.19197178741145));
#14790=CARTESIAN_POINT('Ctrl Pts',(21.2433410956421,-5.70863128218638,7.47569272702411));
#14791=CARTESIAN_POINT('Ctrl Pts',(21.4935141130515,-3.99107778358669,5.6887303718073));
#14792=CARTESIAN_POINT('Ctrl Pts',(21.6168550679505,-3.3148092474812,4.63439611874689));
#14793=CARTESIAN_POINT('Ctrl Pts',(21.8605525202926,-2.424049175255,2.37178196627815));
#14794=CARTESIAN_POINT('Ctrl Pts',(21.9822771983424,-2.2,1.19121278276015));
#14795=CARTESIAN_POINT('Ctrl Pts',(22.1,-2.2,1.66533453693773E-15));
#14796=CARTESIAN_POINT('',(25.9,-2.20000000000001,-1.38777878078145E-14));
#14797=CARTESIAN_POINT('',(78.0000000000001,-2.19999999999999,-1.38777878078145E-14));
#14798=CARTESIAN_POINT('Ctrl Pts',(25.9,-2.2,-1.26287869051112E-14));
#14799=CARTESIAN_POINT('Ctrl Pts',(25.8320584301578,-2.2,0.687486751395677));
#14800=CARTESIAN_POINT('Ctrl Pts',(25.7626425064763,-2.27462673223733,1.37285912097331));
#14801=CARTESIAN_POINT('Ctrl Pts',(25.6232454680745,-2.57052382279369,2.71585246112393));
#14802=CARTESIAN_POINT('Ctrl Pts',(25.5536591008349,-2.79107732111416,3.36964268186213));
#14803=CARTESIAN_POINT('Ctrl Pts',(25.3619357157689,-3.60400801504387,5.12410600030646));
#14804=CARTESIAN_POINT('Ctrl Pts',(25.2353260823093,-4.34505010391429,6.14065935137735));
#14805=CARTESIAN_POINT('Ctrl Pts',(24.9861739757012,-6.17366151377811,7.82617419694253));
#14806=CARTESIAN_POINT('Ctrl Pts',(24.8627326460084,-7.24203907542681,8.48033707933684));
#14807=CARTESIAN_POINT('Ctrl Pts',(24.612591160184,-9.56702001222319,9.33986229220453));
#14808=CARTESIAN_POINT('Ctrl Pts',(24.4911293307759,-10.801000518419,9.53803958026865));
#14809=CARTESIAN_POINT('Ctrl Pts',(24.2403562347155,-13.2749008689799,9.44993444082386));
#14810=CARTESIAN_POINT('Ctrl Pts',(24.1195868569151,-14.4912108845082,9.16464314019057));
#14811=CARTESIAN_POINT('Ctrl Pts',(23.868565051285,-16.7477137680785,8.14290619632623));
#14812=CARTESIAN_POINT('Ctrl Pts',(23.7471727049711,-17.7660153225652,7.41552521022505));
#14813=CARTESIAN_POINT('Ctrl Pts',(23.4962929725926,-19.468575729199,5.60768898329955));
#14814=CARTESIAN_POINT('Ctrl Pts',(23.3730265024687,-20.1352887413488,4.54344435292872));
#14815=CARTESIAN_POINT('Ctrl Pts',(23.132091158415,-20.9895203441915,2.3004420205563));
#14816=CARTESIAN_POINT('Ctrl Pts',(23.0141053600769,-21.2,1.15460863648514));
#14817=CARTESIAN_POINT('Ctrl Pts',(22.9,-21.2,-3.81361608958741E-13));
#14818=CARTESIAN_POINT('Origin',(-58.,-11.7,0.));
#14819=CARTESIAN_POINT('',(-57.5,-19.2,-4.38793205131413E-15));
#14820=CARTESIAN_POINT('',(-57.5,-11.7,7.5));
#14821=CARTESIAN_POINT('Origin',(-57.5,-11.7,-6.93889390390723E-15));
#14822=CARTESIAN_POINT('Origin',(-57.5,-11.7,-6.93889390390723E-15));
#14823=CARTESIAN_POINT('',(-58.,-11.7,7.));
#14824=CARTESIAN_POINT('',(-58.,-11.7,7.));
#14825=CARTESIAN_POINT('Origin',(-58.,-11.7,0.));
#14826=CARTESIAN_POINT('Origin',(78.0000000000001,-11.7,-3.46944695195361E-15));
#14827=CARTESIAN_POINT('',(108.,-4.37815767719625,-1.62500000000001));
#14828=CARTESIAN_POINT('',(108.,-4.37815767719625,1.625));
#14829=CARTESIAN_POINT('Origin',(108.,-11.7,0.));
#14830=CARTESIAN_POINT('',(128.,-4.37815767719625,-1.625));
#14831=CARTESIAN_POINT('',(78.0000000000001,-4.37815767719626,-1.625));
#14832=CARTESIAN_POINT('',(128.,-19.2,-4.38793205131413E-15));
#14833=CARTESIAN_POINT('Origin',(128.,-11.7,-3.46944695195361E-15));
#14834=CARTESIAN_POINT('',(57.,-19.2,-4.38793205131413E-15));
#14835=CARTESIAN_POINT('',(78.0000000000001,-19.2,-4.38793205131413E-15));
#14836=CARTESIAN_POINT('Origin',(57.,-11.7,0.));
#14837=CARTESIAN_POINT('',(128.,-4.37815767719625,1.62499999999998));
#14838=CARTESIAN_POINT('Origin',(128.,-11.7,-3.46944695195361E-15));
#14839=CARTESIAN_POINT('',(78.,-4.37815767719627,1.62500000000001));
#14840=CARTESIAN_POINT('Origin',(78.0000000000001,-11.7,-3.46944695195361E-15));
#14841=CARTESIAN_POINT('',(57.,-19.7,-4.4491643912715E-15));
#14842=CARTESIAN_POINT('Origin',(57.,-11.7,0.));
#14843=CARTESIAN_POINT('',(28.,-19.7,-4.4491643912715E-15));
#14844=CARTESIAN_POINT('',(78.0000000000001,-19.7,-4.4491643912715E-15));
#14845=CARTESIAN_POINT('Origin',(28.,-11.7,-6.93889390390723E-15));
#14846=CARTESIAN_POINT('Origin',(78.0000000000001,-11.7,-3.46944695195361E-15));
#14847=CARTESIAN_POINT('',(-28.,-19.2,-4.38793205131413E-15));
#14848=CARTESIAN_POINT('Origin',(-28.,-11.7,-1.38777878078145E-14));
#14849=CARTESIAN_POINT('',(78.0000000000001,-19.2,-4.38793205131413E-15));
#14850=CARTESIAN_POINT('Origin',(78.0000000000001,-11.7,-3.46944695195361E-15));
#14851=CARTESIAN_POINT('Ctrl Pts',(16.9,-21.2,-8.2367941628566E-30));
#14852=CARTESIAN_POINT('Ctrl Pts',(16.8969830453883,-21.2,-0.0305279423179098));
#14853=CARTESIAN_POINT('Ctrl Pts',(16.8939621685952,-21.1998528492312,-0.061061986178079));
#14854=CARTESIAN_POINT('Ctrl Pts',(16.767248128974,-21.1875162370895,-1.34043950276093));
#14855=CARTESIAN_POINT('Ctrl Pts',(16.6394486076613,-20.9293291909709,-2.57468702777392));
#14856=CARTESIAN_POINT('Ctrl Pts',(16.390901029389,-19.9527852055101,-4.86679898715219));
#14857=CARTESIAN_POINT('Ctrl Pts',(16.2661865852166,-19.2459958496646,-5.90361775701915));
#14858=CARTESIAN_POINT('Ctrl Pts',(16.0164434579476,-17.4760938667979,-7.64340926548421));
#14859=CARTESIAN_POINT('Ctrl Pts',(15.8942543732133,-16.4310772867914,-8.33076824399945));
#14860=CARTESIAN_POINT('Ctrl Pts',(15.643716791377,-14.1377024264444,-9.26493007649783));
#14861=CARTESIAN_POINT('Ctrl Pts',(15.5228012264078,-12.9114457325454,-9.50334490259741));
#14862=CARTESIAN_POINT('Ctrl Pts',(15.2718422511462,-10.4357116660552,-9.49658163777804));
#14863=CARTESIAN_POINT('Ctrl Pts',(15.1508875962576,-9.20987735813006,-9.25110322734291));
#14864=CARTESIAN_POINT('Ctrl Pts',(14.8998967426513,-6.91855760852242,-8.30236799838266));
#14865=CARTESIAN_POINT('Ctrl Pts',(14.7776129198827,-5.87549075136839,-7.60702303698612));
#14866=CARTESIAN_POINT('Ctrl Pts',(14.5269765839982,-4.11220036693074,-5.85068851113425));
#14867=CARTESIAN_POINT('Ctrl Pts',(14.402176887142,-3.41051525358193,-4.80513228098754));
#14868=CARTESIAN_POINT('Ctrl Pts',(14.152310008838,-2.4484427730648,-2.49636756975503));
#14869=CARTESIAN_POINT('Ctrl Pts',(14.023965795097,-2.2,-1.25438434751197));
#14870=CARTESIAN_POINT('Ctrl Pts',(13.7760812749615,-2.2,1.253908055286));
#14871=CARTESIAN_POINT('Ctrl Pts',(13.6477361899215,-2.44826489212498,2.495940694187));
#14872=CARTESIAN_POINT('Ctrl Pts',(13.397823112858,-3.41051525358195,4.8051322809876));
#14873=CARTESIAN_POINT('Ctrl Pts',(13.2730234160018,-4.11220036693081,5.8506885111343));
#14874=CARTESIAN_POINT('Ctrl Pts',(13.0223870801173,-5.87549075136832,7.60702303698604));
#14875=CARTESIAN_POINT('Ctrl Pts',(12.9001032573487,-6.91855760852222,8.30236799838261));
#14876=CARTESIAN_POINT('Ctrl Pts',(12.6491124037424,-9.20987735813006,9.25110322734295));
#14877=CARTESIAN_POINT('Ctrl Pts',(12.5281577488538,-10.4357116660552,9.49658163777806));
#14878=CARTESIAN_POINT('Ctrl Pts',(12.2771987735922,-12.9114457325453,9.50334490259743));
#14879=CARTESIAN_POINT('Ctrl Pts',(12.156283208623,-14.1377024264444,9.26493007649789));
#14880=CARTESIAN_POINT('Ctrl Pts',(11.9057456267867,-16.4310772867913,8.33076824399952));
#14881=CARTESIAN_POINT('Ctrl Pts',(11.7835565420523,-17.4760938667978,7.64340926548429));
#14882=CARTESIAN_POINT('Ctrl Pts',(11.5338134147833,-19.2459958496645,5.90361775701927));
#14883=CARTESIAN_POINT('Ctrl Pts',(11.4090989706109,-19.9527852055101,4.86679898715229));
#14884=CARTESIAN_POINT('Ctrl Pts',(11.1605513923387,-20.929329190971,2.574687027774));
#14885=CARTESIAN_POINT('Ctrl Pts',(11.032751871026,-21.1875162370896,1.340439502761));
#14886=CARTESIAN_POINT('Ctrl Pts',(10.9060378314048,-21.1998528492313,0.0610619861781323));
#14887=CARTESIAN_POINT('Ctrl Pts',(10.9030169546117,-21.2,0.0305279423179378));
#14888=CARTESIAN_POINT('Ctrl Pts',(10.9,-21.2,6.20405247894856E-15));
#14889=CARTESIAN_POINT('Ctrl Pts',(13.1000000000002,-21.2,1.5694563704205E-12));
#14890=CARTESIAN_POINT('Ctrl Pts',(13.1150618716887,-21.2,0.152407977343253));
#14891=CARTESIAN_POINT('Ctrl Pts',(13.1302184694214,-21.1963324367572,0.304937370638801));
#14892=CARTESIAN_POINT('Ctrl Pts',(13.2700599843257,-21.1288573016021,1.70456409769737));
#14893=CARTESIAN_POINT('Ctrl Pts',(13.3978280547826,-20.8234635749735,2.92771876120427));
#14894=CARTESIAN_POINT('Ctrl Pts',(13.6454592566918,-19.755260072567,5.18963741030103));
#14895=CARTESIAN_POINT('Ctrl Pts',(13.7732390331541,-19.0012386404909,6.20590007975632));
#14896=CARTESIAN_POINT('Ctrl Pts',(14.0232777368833,-17.1471853740769,7.88231274196907));
#14897=CARTESIAN_POINT('Ctrl Pts',(14.1476486571035,-16.0673203360107,8.52815677935463));
#14898=CARTESIAN_POINT('Ctrl Pts',(14.3983590751342,-13.7248517892438,9.36430425037921));
#14899=CARTESIAN_POINT('Ctrl Pts',(14.520375998781,-12.4854983155022,9.54845471360794));
#14900=CARTESIAN_POINT('Ctrl Pts',(14.7713863912166,-10.0092570137193,9.42996830424106));
#14901=CARTESIAN_POINT('Ctrl Pts',(14.8922543670058,-8.79600881109443,9.1296032176108));
#14902=CARTESIAN_POINT('Ctrl Pts',(15.1431766592368,-6.55370184479103,8.08065075646646));
#14903=CARTESIAN_POINT('Ctrl Pts',(15.2641950892462,-5.54595419660828,7.34228914700703));
#14904=CARTESIAN_POINT('Ctrl Pts',(15.5146409061442,-3.86915103688522,5.51938731615909));
#14905=CARTESIAN_POINT('Ctrl Pts',(15.6371179553,-3.21662243900297,4.4517706334838));
#14906=CARTESIAN_POINT('Ctrl Pts',(15.8867179619448,-2.35695918963997,2.12233210287465));
#14907=CARTESIAN_POINT('Ctrl Pts',(16.0118911216994,-2.15969596306437,0.882356458430438));
#14908=CARTESIAN_POINT('Ctrl Pts',(16.2602345530853,-2.25420339436364,-1.60900886831394));
#14909=CARTESIAN_POINT('Ctrl Pts',(16.3881490721731,-2.5475691743667,-2.8363907156804));
#14910=CARTESIAN_POINT('Ctrl Pts',(16.6362896776214,-3.59330951586658,-5.10859098415954));
#14911=CARTESIAN_POINT('Ctrl Pts',(16.7633666485782,-4.33619714865433,-6.13122431775599));
#14912=CARTESIAN_POINT('Ctrl Pts',(17.0135568268943,-6.17095257434411,-7.82493779010911));
#14913=CARTESIAN_POINT('Ctrl Pts',(17.1374069120597,-7.24301853066505,-8.48147631282628));
#14914=CARTESIAN_POINT('Ctrl Pts',(17.3882015412574,-9.57470582039923,-9.34192598080633));
#14915=CARTESIAN_POINT('Ctrl Pts',(17.5099110598593,-10.8112640706003,-9.53930664709422));
#14916=CARTESIAN_POINT('Ctrl Pts',(17.7609348528615,-13.2876375702419,-9.44783485576954));
#14917=CARTESIAN_POINT('Ctrl Pts',(17.8817307023484,-14.5038018029798,-9.16083147073306));
#14918=CARTESIAN_POINT('Ctrl Pts',(18.1325938901276,-16.7573768406909,-8.13662124256136));
#14919=CARTESIAN_POINT('Ctrl Pts',(18.2537849940001,-17.7732966317507,-7.40924768217617));
#14920=CARTESIAN_POINT('Ctrl Pts',(18.5041011927066,-19.4704623912838,-5.60421999604294));
#14921=CARTESIAN_POINT('Ctrl Pts',(18.6269875482744,-20.1348513062228,-4.54320233464012));
#14922=CARTESIAN_POINT('Ctrl Pts',(18.8676457342621,-20.9890409731633,-2.30299493605579));
#14923=CARTESIAN_POINT('Ctrl Pts',(18.9857650877243,-21.2,-1.15591954850146));
#14924=CARTESIAN_POINT('Ctrl Pts',(19.1,-21.2,3.13915560212763E-13));
#14925=CARTESIAN_POINT('Origin',(-28.,-4.2,-6.93889390390723E-15));
#14926=CARTESIAN_POINT('Origin',(28.,-2.2,3.46944695195361E-15));
#14927=CARTESIAN_POINT('Origin',(57.,-3.69999999999999,-2.08166817117217E-14));
#14928=CARTESIAN_POINT('Origin',(24.,2.3,-3.46944695195361E-15));
#14929=CARTESIAN_POINT('',(24.9704939903643,1.5411253090549,0.));
#14930=CARTESIAN_POINT('',(25.4352469951821,-0.329437345472555,0.));
#14931=CARTESIAN_POINT('',(23.0295060096357,1.5411253090549,0.));
#14932=CARTESIAN_POINT('',(22.5647530048179,-0.329437345472541,-2.08166817117217E-14));
#14933=CARTESIAN_POINT('Origin',(24.,1.3,-6.93889390390723E-15));
#14934=CARTESIAN_POINT('Ctrl Pts',(-0.97049399036428,1.5411253090549,-6.93889390390723E-15));
#14935=CARTESIAN_POINT('Ctrl Pts',(-0.756208276078568,1.5411253090549,-3.02220044537404));
#14936=CARTESIAN_POINT('Ctrl Pts',(-0.541922561792853,0.229841679453259,
-5.74510895921687));
#14937=CARTESIAN_POINT('Ctrl Pts',(-0.327636847507138,-1.08144195014838,
-8.4680174730597));
#14938=CARTESIAN_POINT('Ctrl Pts',(-0.113351133221425,-3.4442934046707,
-10.3523286299233));
#14939=CARTESIAN_POINT('Ctrl Pts',(0.100934581064289,-5.80714485919302,
-12.236639786787));
#14940=CARTESIAN_POINT('Ctrl Pts',(0.315220295350005,-8.75357242959651,
-12.9091426524948));
#14941=CARTESIAN_POINT('Ctrl Pts',(0.529506009635718,-11.7,-13.5816455182026));
#14942=CARTESIAN_POINT('Ctrl Pts',(0.743791723921435,-14.6464275704035,
-12.9091426524948));
#14943=CARTESIAN_POINT('Ctrl Pts',(0.958077438207147,-17.592855140807,-12.236639786787));
#14944=CARTESIAN_POINT('Ctrl Pts',(1.17236315249286,-19.9557065953293,-10.3523286299233));
#14945=CARTESIAN_POINT('Ctrl Pts',(1.38664886677857,-22.3185580498516,-8.4680174730597));
#14946=CARTESIAN_POINT('Ctrl Pts',(1.60093458106429,-23.6298416794532,-5.74510895921687));
#14947=CARTESIAN_POINT('Ctrl Pts',(1.81522029535,-24.9411253090549,-3.02220044537404));
#14948=CARTESIAN_POINT('Ctrl Pts',(2.02950600963572,-24.9411253090549,6.93889390390723E-15));
#14949=CARTESIAN_POINT('Ctrl Pts',(2.24379172392143,-24.9411253090549,3.02220044537403));
#14950=CARTESIAN_POINT('Ctrl Pts',(2.45807743820715,-23.6298416794532,5.74510895921686));
#14951=CARTESIAN_POINT('Ctrl Pts',(2.67236315249286,-22.3185580498516,8.4680174730597));
#14952=CARTESIAN_POINT('Ctrl Pts',(2.88664886677858,-19.9557065953293,10.3523286299233));
#14953=CARTESIAN_POINT('Ctrl Pts',(3.10093458106429,-17.592855140807,12.236639786787));
#14954=CARTESIAN_POINT('Ctrl Pts',(3.31522029535001,-14.6464275704035,12.9091426524948));
#14955=CARTESIAN_POINT('Ctrl Pts',(3.52950600963572,-11.7,13.5816455182026));
#14956=CARTESIAN_POINT('Ctrl Pts',(3.74379172392143,-8.7535724295965,12.9091426524948));
#14957=CARTESIAN_POINT('Ctrl Pts',(3.95807743820715,-5.80714485919301,12.236639786787));
#14958=CARTESIAN_POINT('Ctrl Pts',(4.17236315249286,-3.4442934046707,10.3523286299233));
#14959=CARTESIAN_POINT('Ctrl Pts',(4.38664886677858,-1.08144195014837,8.46801747305969));
#14960=CARTESIAN_POINT('Ctrl Pts',(4.60093458106429,0.229841679453252,5.74510895921686));
#14961=CARTESIAN_POINT('Ctrl Pts',(4.81522029535,1.5411253090549,3.02220044537404));
#14962=CARTESIAN_POINT('Ctrl Pts',(5.02950600963572,1.5411253090549,0.));
#14963=CARTESIAN_POINT('Ctrl Pts',(5.24379172392143,1.5411253090549,-3.02220044537404));
#14964=CARTESIAN_POINT('Ctrl Pts',(5.45807743820715,0.229841679453252,-5.74510895921687));
#14965=CARTESIAN_POINT('Ctrl Pts',(5.67236315249286,-1.08144195014837,-8.4680174730597));
#14966=CARTESIAN_POINT('Ctrl Pts',(5.88664886677858,-3.4442934046707,-10.3523286299233));
#14967=CARTESIAN_POINT('Ctrl Pts',(6.10093458106429,-5.80714485919301,-12.236639786787));
#14968=CARTESIAN_POINT('Ctrl Pts',(6.31522029535001,-8.75357242959651,-12.9091426524948));
#14969=CARTESIAN_POINT('Ctrl Pts',(6.52950600963572,-11.7,-13.5816455182026));
#14970=CARTESIAN_POINT('Ctrl Pts',(6.74379172392144,-14.6464275704035,-12.9091426524948));
#14971=CARTESIAN_POINT('Ctrl Pts',(6.95807743820715,-17.592855140807,-12.236639786787));
#14972=CARTESIAN_POINT('Ctrl Pts',(7.17236315249286,-19.9557065953293,-10.3523286299233));
#14973=CARTESIAN_POINT('Ctrl Pts',(7.38664886677858,-22.3185580498516,-8.4680174730597));
#14974=CARTESIAN_POINT('Ctrl Pts',(7.60093458106429,-23.6298416794532,-5.74510895921687));
#14975=CARTESIAN_POINT('Ctrl Pts',(7.81522029535,-24.9411253090549,-3.02220044537404));
#14976=CARTESIAN_POINT('Ctrl Pts',(8.02950600963572,-24.9411253090549,-6.93889390390723E-15));
#14977=CARTESIAN_POINT('Ctrl Pts',(8.24379172392143,-24.9411253090549,3.02220044537402));
#14978=CARTESIAN_POINT('Ctrl Pts',(8.45807743820715,-23.6298416794532,5.74510895921685));
#14979=CARTESIAN_POINT('Ctrl Pts',(8.67236315249286,-22.3185580498516,8.4680174730597));
#14980=CARTESIAN_POINT('Ctrl Pts',(8.88664886677858,-19.9557065953293,10.3523286299233));
#14981=CARTESIAN_POINT('Ctrl Pts',(9.10093458106429,-17.592855140807,12.236639786787));
#14982=CARTESIAN_POINT('Ctrl Pts',(9.31522029535001,-14.6464275704035,12.9091426524948));
#14983=CARTESIAN_POINT('Ctrl Pts',(9.52950600963572,-11.7,13.5816455182026));
#14984=CARTESIAN_POINT('Ctrl Pts',(9.74379172392144,-8.75357242959651,12.9091426524948));
#14985=CARTESIAN_POINT('Ctrl Pts',(9.95807743820714,-5.80714485919302,12.236639786787));
#14986=CARTESIAN_POINT('Ctrl Pts',(10.1723631524929,-3.4442934046707,10.3523286299233));
#14987=CARTESIAN_POINT('Ctrl Pts',(10.3866488667786,-1.08144195014837,8.4680174730597));
#14988=CARTESIAN_POINT('Ctrl Pts',(10.6009345810643,0.229841679453252,5.74510895921686));
#14989=CARTESIAN_POINT('Ctrl Pts',(10.81522029535,1.5411253090549,3.02220044537402));
#14990=CARTESIAN_POINT('Ctrl Pts',(11.0295060096357,1.5411253090549,6.93889390390723E-15));
#14991=CARTESIAN_POINT('Ctrl Pts',(11.2437917239214,1.54112530905489,-3.02220044537404));
#14992=CARTESIAN_POINT('Ctrl Pts',(11.4580774382071,0.229841679453259,-5.74510895921686));
#14993=CARTESIAN_POINT('Ctrl Pts',(11.6723631524929,-1.08144195014837,-8.4680174730597));
#14994=CARTESIAN_POINT('Ctrl Pts',(11.8866488667786,-3.4442934046707,-10.3523286299233));
#14995=CARTESIAN_POINT('Ctrl Pts',(12.1009345810643,-5.80714485919302,-12.236639786787));
#14996=CARTESIAN_POINT('Ctrl Pts',(12.31522029535,-8.75357242959649,-12.9091426524948));
#14997=CARTESIAN_POINT('Ctrl Pts',(12.5295060096357,-11.7,-13.5816455182026));
#14998=CARTESIAN_POINT('Ctrl Pts',(12.7437917239214,-14.6464275704035,-12.9091426524948));
#14999=CARTESIAN_POINT('Ctrl Pts',(12.9580774382071,-17.592855140807,-12.236639786787));
#15000=CARTESIAN_POINT('Ctrl Pts',(13.1723631524929,-19.9557065953293,-10.3523286299233));
#15001=CARTESIAN_POINT('Ctrl Pts',(13.3866488667786,-22.3185580498516,-8.4680174730597));
#15002=CARTESIAN_POINT('Ctrl Pts',(13.6009345810643,-23.6298416794532,-5.74510895921687));
#15003=CARTESIAN_POINT('Ctrl Pts',(13.81522029535,-24.9411253090549,-3.02220044537403));
#15004=CARTESIAN_POINT('Ctrl Pts',(14.0295060096357,-24.9411253090549,-6.93889390390723E-15));
#15005=CARTESIAN_POINT('Ctrl Pts',(14.2437917239214,-24.9411253090549,3.02220044537403));
#15006=CARTESIAN_POINT('Ctrl Pts',(14.4580774382072,-23.6298416794532,5.74510895921685));
#15007=CARTESIAN_POINT('Ctrl Pts',(14.6723631524929,-22.3185580498516,8.46801747305969));
#15008=CARTESIAN_POINT('Ctrl Pts',(14.8866488667786,-19.9557065953293,10.3523286299233));
#15009=CARTESIAN_POINT('Ctrl Pts',(15.1009345810643,-17.592855140807,12.236639786787));
#15010=CARTESIAN_POINT('Ctrl Pts',(15.31522029535,-14.6464275704035,12.9091426524948));
#15011=CARTESIAN_POINT('Ctrl Pts',(15.5295060096357,-11.7,13.5816455182026));
#15012=CARTESIAN_POINT('Ctrl Pts',(15.7437917239214,-8.75357242959651,12.9091426524948));
#15013=CARTESIAN_POINT('Ctrl Pts',(15.9580774382071,-5.80714485919302,12.236639786787));
#15014=CARTESIAN_POINT('Ctrl Pts',(16.1723631524929,-3.4442934046707,10.3523286299233));
#15015=CARTESIAN_POINT('Ctrl Pts',(16.3866488667786,-1.08144195014837,8.46801747305969));
#15016=CARTESIAN_POINT('Ctrl Pts',(16.6009345810643,0.229841679453266,5.74510895921686));
#15017=CARTESIAN_POINT('Ctrl Pts',(16.81522029535,1.5411253090549,3.02220044537404));
#15018=CARTESIAN_POINT('Ctrl Pts',(17.0295060096357,1.5411253090549,-2.08166817117217E-14));
#15019=CARTESIAN_POINT('Ctrl Pts',(17.2437917239214,1.5411253090549,-3.02220044537405));
#15020=CARTESIAN_POINT('Ctrl Pts',(17.4580774382072,0.229841679453266,-5.74510895921688));
#15021=CARTESIAN_POINT('Ctrl Pts',(17.6723631524929,-1.08144195014837,-8.46801747305971));
#15022=CARTESIAN_POINT('Ctrl Pts',(17.8866488667786,-3.44429340467071,-10.3523286299233));
#15023=CARTESIAN_POINT('Ctrl Pts',(18.1009345810643,-5.80714485919302,-12.236639786787));
#15024=CARTESIAN_POINT('Ctrl Pts',(18.31522029535,-8.75357242959651,-12.9091426524948));
#15025=CARTESIAN_POINT('Ctrl Pts',(18.5295060096357,-11.7,-13.5816455182026));
#15026=CARTESIAN_POINT('Ctrl Pts',(18.7437917239214,-14.6464275704035,-12.9091426524948));
#15027=CARTESIAN_POINT('Ctrl Pts',(18.9580774382071,-17.592855140807,-12.236639786787));
#15028=CARTESIAN_POINT('Ctrl Pts',(19.1723631524929,-19.9557065953293,-10.3523286299233));
#15029=CARTESIAN_POINT('Ctrl Pts',(19.3866488667786,-22.3185580498516,-8.4680174730597));
#15030=CARTESIAN_POINT('Ctrl Pts',(19.6009345810643,-23.6298416794532,-5.74510895921687));
#15031=CARTESIAN_POINT('Ctrl Pts',(19.81522029535,-24.9411253090549,-3.02220044537404));
#15032=CARTESIAN_POINT('Ctrl Pts',(20.0295060096357,-24.9411253090549,0.));
#15033=CARTESIAN_POINT('Ctrl Pts',(20.2437917239214,-24.9411253090549,3.02220044537403));
#15034=CARTESIAN_POINT('Ctrl Pts',(20.4580774382071,-23.6298416794532,5.74510895921685));
#15035=CARTESIAN_POINT('Ctrl Pts',(20.6723631524929,-22.3185580498516,8.46801747305969));
#15036=CARTESIAN_POINT('Ctrl Pts',(20.8866488667786,-19.9557065953293,10.3523286299233));
#15037=CARTESIAN_POINT('Ctrl Pts',(21.1009345810643,-17.5928551408069,12.236639786787));
#15038=CARTESIAN_POINT('Ctrl Pts',(21.31522029535,-14.6464275704035,12.9091426524948));
#15039=CARTESIAN_POINT('Ctrl Pts',(21.5295060096357,-11.7,13.5816455182026));
#15040=CARTESIAN_POINT('Ctrl Pts',(21.7437917239214,-8.75357242959651,12.9091426524948));
#15041=CARTESIAN_POINT('Ctrl Pts',(21.9580774382071,-5.80714485919301,12.236639786787));
#15042=CARTESIAN_POINT('Ctrl Pts',(22.1723631524929,-3.4442934046707,10.3523286299233));
#15043=CARTESIAN_POINT('Ctrl Pts',(22.3866488667786,-1.08144195014837,8.4680174730597));
#15044=CARTESIAN_POINT('Ctrl Pts',(22.6009345810643,0.229841679453259,5.74510895921686));
#15045=CARTESIAN_POINT('Ctrl Pts',(22.81522029535,1.54112530905491,3.02220044537404));
#15046=CARTESIAN_POINT('Ctrl Pts',(23.0295060096357,1.5411253090549,0.));
#15047=CARTESIAN_POINT('Ctrl Pts',(-1.9,-2.2,0.));
#15048=CARTESIAN_POINT('Ctrl Pts',(-1.68571428571429,-2.19999999999999,
-2.16831300670641));
#15049=CARTESIAN_POINT('Ctrl Pts',(-1.47142857142857,-3.14079575492701,
-4.1218955216168));
#15050=CARTESIAN_POINT('Ctrl Pts',(-1.25714285714286,-4.08159150985404,
-6.07547803652718));
#15051=CARTESIAN_POINT('Ctrl Pts',(-1.04285714285715,-5.77684688234203,
-7.42739908344627));
#15052=CARTESIAN_POINT('Ctrl Pts',(-0.828571428571431,-7.47210225483002,
-8.77932013036538));
#15053=CARTESIAN_POINT('Ctrl Pts',(-0.614285714285715,-9.58605112741501,
-9.26181516572732));
#15054=CARTESIAN_POINT('Ctrl Pts',(-0.400000000000003,-11.7,-9.74431020108925));
#15055=CARTESIAN_POINT('Ctrl Pts',(-0.185714285714288,-13.813948872585,
-9.26181516572733));
#15056=CARTESIAN_POINT('Ctrl Pts',(0.0285714285714265,-15.92789774517,-8.7793201303654));
#15057=CARTESIAN_POINT('Ctrl Pts',(0.242857142857143,-17.6231531176579,
-7.42739908344628));
#15058=CARTESIAN_POINT('Ctrl Pts',(0.457142857142854,-19.3184084901459,
-6.07547803652718));
#15059=CARTESIAN_POINT('Ctrl Pts',(0.671428571428569,-20.259204245073,-4.1218955216168));
#15060=CARTESIAN_POINT('Ctrl Pts',(0.885714285714283,-21.2,-2.16831300670643));
#15061=CARTESIAN_POINT('Ctrl Pts',(1.1,-21.2,-6.93889390390723E-15));
#15062=CARTESIAN_POINT('Ctrl Pts',(1.31428571428571,-21.2,2.16831300670641));
#15063=CARTESIAN_POINT('Ctrl Pts',(1.52857142857143,-20.259204245073,4.1218955216168));
#15064=CARTESIAN_POINT('Ctrl Pts',(1.74285714285714,-19.318408490146,6.07547803652716));
#15065=CARTESIAN_POINT('Ctrl Pts',(1.95714285714286,-17.623153117658,7.42739908344628));
#15066=CARTESIAN_POINT('Ctrl Pts',(2.17142857142857,-15.92789774517,8.77932013036537));
#15067=CARTESIAN_POINT('Ctrl Pts',(2.38571428571428,-13.813948872585,9.26181516572731));
#15068=CARTESIAN_POINT('Ctrl Pts',(2.6,-11.7,9.74431020108925));
#15069=CARTESIAN_POINT('Ctrl Pts',(2.81428571428571,-9.586051127415,9.26181516572731));
#15070=CARTESIAN_POINT('Ctrl Pts',(3.02857142857143,-7.47210225483002,8.77932013036537));
#15071=CARTESIAN_POINT('Ctrl Pts',(3.24285714285714,-5.77684688234203,7.42739908344628));
#15072=CARTESIAN_POINT('Ctrl Pts',(3.45714285714285,-4.08159150985404,6.07547803652717));
#15073=CARTESIAN_POINT('Ctrl Pts',(3.67142857142857,-3.14079575492702,4.1218955216168));
#15074=CARTESIAN_POINT('Ctrl Pts',(3.88571428571428,-2.2,2.16831300670642));
#15075=CARTESIAN_POINT('Ctrl Pts',(4.1,-2.20000000000001,-6.93889390390723E-15));
#15076=CARTESIAN_POINT('Ctrl Pts',(4.31428571428571,-2.19999999999999,-2.16831300670641));
#15077=CARTESIAN_POINT('Ctrl Pts',(4.52857142857143,-3.14079575492703,-4.1218955216168));
#15078=CARTESIAN_POINT('Ctrl Pts',(4.74285714285714,-4.08159150985404,-6.07547803652716));
#15079=CARTESIAN_POINT('Ctrl Pts',(4.95714285714286,-5.77684688234202,-7.42739908344627));
#15080=CARTESIAN_POINT('Ctrl Pts',(5.17142857142857,-7.47210225483002,-8.77932013036537));
#15081=CARTESIAN_POINT('Ctrl Pts',(5.38571428571428,-9.58605112741501,-9.26181516572731));
#15082=CARTESIAN_POINT('Ctrl Pts',(5.6,-11.7,-9.74431020108925));
#15083=CARTESIAN_POINT('Ctrl Pts',(5.81428571428571,-13.813948872585,-9.26181516572731));
#15084=CARTESIAN_POINT('Ctrl Pts',(6.02857142857142,-15.92789774517,-8.77932013036537));
#15085=CARTESIAN_POINT('Ctrl Pts',(6.24285714285714,-17.623153117658,-7.42739908344628));
#15086=CARTESIAN_POINT('Ctrl Pts',(6.45714285714286,-19.3184084901459,-6.07547803652718));
#15087=CARTESIAN_POINT('Ctrl Pts',(6.67142857142857,-20.259204245073,-4.12189552161681));
#15088=CARTESIAN_POINT('Ctrl Pts',(6.88571428571428,-21.2,-2.16831300670643));
#15089=CARTESIAN_POINT('Ctrl Pts',(7.1,-21.2,-1.04083408558608E-14));
#15090=CARTESIAN_POINT('Ctrl Pts',(7.31428571428571,-21.2,2.16831300670641));
#15091=CARTESIAN_POINT('Ctrl Pts',(7.52857142857143,-20.259204245073,4.12189552161679));
#15092=CARTESIAN_POINT('Ctrl Pts',(7.74285714285714,-19.3184084901459,6.07547803652717));
#15093=CARTESIAN_POINT('Ctrl Pts',(7.95714285714285,-17.623153117658,7.42739908344627));
#15094=CARTESIAN_POINT('Ctrl Pts',(8.17142857142857,-15.92789774517,8.77932013036537));
#15095=CARTESIAN_POINT('Ctrl Pts',(8.38571428571429,-13.813948872585,9.26181516572731));
#15096=CARTESIAN_POINT('Ctrl Pts',(8.6,-11.7,9.74431020108926));
#15097=CARTESIAN_POINT('Ctrl Pts',(8.81428571428571,-9.58605112741501,9.26181516572732));
#15098=CARTESIAN_POINT('Ctrl Pts',(9.02857142857143,-7.47210225483001,8.77932013036537));
#15099=CARTESIAN_POINT('Ctrl Pts',(9.24285714285714,-5.77684688234203,7.42739908344627));
#15100=CARTESIAN_POINT('Ctrl Pts',(9.45714285714285,-4.08159150985402,6.07547803652717));
#15101=CARTESIAN_POINT('Ctrl Pts',(9.67142857142857,-3.14079575492703,4.12189552161679));
#15102=CARTESIAN_POINT('Ctrl Pts',(9.88571428571429,-2.20000000000001,2.16831300670642));
#15103=CARTESIAN_POINT('Ctrl Pts',(10.1,-2.19999999999999,0.));
#15104=CARTESIAN_POINT('Ctrl Pts',(10.3142857142857,-2.2,-2.16831300670643));
#15105=CARTESIAN_POINT('Ctrl Pts',(10.5285714285714,-3.14079575492703,-4.12189552161681));
#15106=CARTESIAN_POINT('Ctrl Pts',(10.7428571428571,-4.08159150985404,-6.07547803652718));
#15107=CARTESIAN_POINT('Ctrl Pts',(10.9571428571429,-5.77684688234203,-7.42739908344627));
#15108=CARTESIAN_POINT('Ctrl Pts',(11.1714285714286,-7.47210225483002,-8.77932013036538));
#15109=CARTESIAN_POINT('Ctrl Pts',(11.3857142857143,-9.58605112741501,-9.26181516572732));
#15110=CARTESIAN_POINT('Ctrl Pts',(11.6,-11.7,-9.74431020108924));
#15111=CARTESIAN_POINT('Ctrl Pts',(11.8142857142857,-13.813948872585,-9.26181516572731));
#15112=CARTESIAN_POINT('Ctrl Pts',(12.0285714285714,-15.92789774517,-8.77932013036537));
#15113=CARTESIAN_POINT('Ctrl Pts',(12.2428571428571,-17.623153117658,-7.42739908344628));
#15114=CARTESIAN_POINT('Ctrl Pts',(12.4571428571429,-19.3184084901459,-6.07547803652717));
#15115=CARTESIAN_POINT('Ctrl Pts',(12.6714285714286,-20.259204245073,-4.1218955216168));
#15116=CARTESIAN_POINT('Ctrl Pts',(12.8857142857143,-21.2,-2.16831300670643));
#15117=CARTESIAN_POINT('Ctrl Pts',(13.1,-21.2,-1.04083408558608E-14));
#15118=CARTESIAN_POINT('Ctrl Pts',(13.3142857142857,-21.2,2.16831300670641));
#15119=CARTESIAN_POINT('Ctrl Pts',(13.5285714285714,-20.259204245073,4.12189552161679));
#15120=CARTESIAN_POINT('Ctrl Pts',(13.7428571428571,-19.3184084901459,6.07547803652717));
#15121=CARTESIAN_POINT('Ctrl Pts',(13.9571428571429,-17.623153117658,7.42739908344627));
#15122=CARTESIAN_POINT('Ctrl Pts',(14.1714285714286,-15.92789774517,8.77932013036537));
#15123=CARTESIAN_POINT('Ctrl Pts',(14.3857142857143,-13.813948872585,9.26181516572731));
#15124=CARTESIAN_POINT('Ctrl Pts',(14.6,-11.7,9.74431020108925));
#15125=CARTESIAN_POINT('Ctrl Pts',(14.8142857142857,-9.58605112741501,9.26181516572731));
#15126=CARTESIAN_POINT('Ctrl Pts',(15.0285714285714,-7.47210225483002,8.77932013036537));
#15127=CARTESIAN_POINT('Ctrl Pts',(15.2428571428571,-5.77684688234202,7.42739908344628));
#15128=CARTESIAN_POINT('Ctrl Pts',(15.4571428571429,-4.08159150985404,6.07547803652717));
#15129=CARTESIAN_POINT('Ctrl Pts',(15.6714285714286,-3.14079575492702,4.1218955216168));
#15130=CARTESIAN_POINT('Ctrl Pts',(15.8857142857143,-2.20000000000001,2.16831300670642));
#15131=CARTESIAN_POINT('Ctrl Pts',(16.1,-2.19999999999999,-6.93889390390723E-15));
#15132=CARTESIAN_POINT('Ctrl Pts',(16.3142857142857,-2.19999999999999,-2.16831300670641));
#15133=CARTESIAN_POINT('Ctrl Pts',(16.5285714285714,-3.14079575492702,-4.1218955216168));
#15134=CARTESIAN_POINT('Ctrl Pts',(16.7428571428571,-4.08159150985404,-6.07547803652718));
#15135=CARTESIAN_POINT('Ctrl Pts',(16.9571428571428,-5.77684688234203,-7.42739908344629));
#15136=CARTESIAN_POINT('Ctrl Pts',(17.1714285714286,-7.47210225483002,-8.77932013036539));
#15137=CARTESIAN_POINT('Ctrl Pts',(17.3857142857143,-9.58605112741501,-9.26181516572732));
#15138=CARTESIAN_POINT('Ctrl Pts',(17.6,-11.7,-9.74431020108926));
#15139=CARTESIAN_POINT('Ctrl Pts',(17.8142857142857,-13.813948872585,-9.2618151657273));
#15140=CARTESIAN_POINT('Ctrl Pts',(18.0285714285714,-15.92789774517,-8.77932013036537));
#15141=CARTESIAN_POINT('Ctrl Pts',(18.2428571428571,-17.6231531176579,-7.42739908344628));
#15142=CARTESIAN_POINT('Ctrl Pts',(18.4571428571428,-19.3184084901459,-6.07547803652718));
#15143=CARTESIAN_POINT('Ctrl Pts',(18.6714285714286,-20.259204245073,-4.1218955216168));
#15144=CARTESIAN_POINT('Ctrl Pts',(18.8857142857143,-21.2,-2.16831300670642));
#15145=CARTESIAN_POINT('Ctrl Pts',(19.1,-21.2,0.));
#15146=CARTESIAN_POINT('Ctrl Pts',(19.3142857142857,-21.2,2.16831300670641));
#15147=CARTESIAN_POINT('Ctrl Pts',(19.5285714285714,-20.259204245073,4.12189552161679));
#15148=CARTESIAN_POINT('Ctrl Pts',(19.7428571428572,-19.318408490146,6.07547803652717));
#15149=CARTESIAN_POINT('Ctrl Pts',(19.9571428571429,-17.623153117658,7.42739908344627));
#15150=CARTESIAN_POINT('Ctrl Pts',(20.1714285714286,-15.92789774517,8.77932013036537));
#15151=CARTESIAN_POINT('Ctrl Pts',(20.3857142857143,-13.813948872585,9.26181516572731));
#15152=CARTESIAN_POINT('Ctrl Pts',(20.6,-11.7,9.74431020108925));
#15153=CARTESIAN_POINT('Ctrl Pts',(20.8142857142857,-9.58605112741501,9.2618151657273));
#15154=CARTESIAN_POINT('Ctrl Pts',(21.0285714285714,-7.47210225483003,8.77932013036538));
#15155=CARTESIAN_POINT('Ctrl Pts',(21.2428571428572,-5.77684688234203,7.42739908344627));
#15156=CARTESIAN_POINT('Ctrl Pts',(21.4571428571429,-4.08159150985404,6.07547803652717));
#15157=CARTESIAN_POINT('Ctrl Pts',(21.6714285714286,-3.14079575492702,4.1218955216168));
#15158=CARTESIAN_POINT('Ctrl Pts',(21.8857142857143,-2.2,2.16831300670641));
#15159=CARTESIAN_POINT('Ctrl Pts',(22.1,-2.2,0.));
#15160=CARTESIAN_POINT('',(-0.97049399036428,1.5411253090549,-6.93889390390723E-15));
#15161=CARTESIAN_POINT('',(-1.43524699518214,-0.329437345472555,0.));
#15162=CARTESIAN_POINT('Ctrl Pts',(-0.97049399036428,1.5411253090549,-6.93889390390723E-15));
#15163=CARTESIAN_POINT('Ctrl Pts',(-0.756208276078568,1.5411253090549,-3.02220044537404));
#15164=CARTESIAN_POINT('Ctrl Pts',(-0.541922561792853,0.229841679453259,
-5.74510895921687));
#15165=CARTESIAN_POINT('Ctrl Pts',(-0.327636847507139,-1.08144195014838,
-8.4680174730597));
#15166=CARTESIAN_POINT('Ctrl Pts',(-0.113351133221425,-3.4442934046707,
-10.3523286299233));
#15167=CARTESIAN_POINT('Ctrl Pts',(0.10093458106429,-5.80714485919302,-12.236639786787));
#15168=CARTESIAN_POINT('Ctrl Pts',(0.315220295350005,-8.75357242959651,
-12.9091426524948));
#15169=CARTESIAN_POINT('Ctrl Pts',(0.529506009635718,-11.7,-13.5816455182026));
#15170=CARTESIAN_POINT('Ctrl Pts',(0.743791723921435,-14.6464275704035,
-12.9091426524948));
#15171=CARTESIAN_POINT('Ctrl Pts',(0.958077438207147,-17.592855140807,-12.236639786787));
#15172=CARTESIAN_POINT('Ctrl Pts',(1.17236315249286,-19.9557065953293,-10.3523286299233));
#15173=CARTESIAN_POINT('Ctrl Pts',(1.38664886677857,-22.3185580498516,-8.4680174730597));
#15174=CARTESIAN_POINT('Ctrl Pts',(1.60093458106429,-23.6298416794532,-5.74510895921687));
#15175=CARTESIAN_POINT('Ctrl Pts',(1.81522029535,-24.9411253090549,-3.02220044537404));
#15176=CARTESIAN_POINT('Ctrl Pts',(2.02950600963572,-24.9411253090549,6.93889390390723E-15));
#15177=CARTESIAN_POINT('Ctrl Pts',(2.24379172392143,-24.9411253090549,3.02220044537403));
#15178=CARTESIAN_POINT('Ctrl Pts',(2.45807743820715,-23.6298416794532,5.74510895921686));
#15179=CARTESIAN_POINT('Ctrl Pts',(2.67236315249286,-22.3185580498516,8.4680174730597));
#15180=CARTESIAN_POINT('Ctrl Pts',(2.88664886677858,-19.9557065953293,10.3523286299233));
#15181=CARTESIAN_POINT('Ctrl Pts',(3.10093458106429,-17.592855140807,12.236639786787));
#15182=CARTESIAN_POINT('Ctrl Pts',(3.31522029535001,-14.6464275704035,12.9091426524948));
#15183=CARTESIAN_POINT('Ctrl Pts',(3.52950600963572,-11.7,13.5816455182026));
#15184=CARTESIAN_POINT('Ctrl Pts',(3.74379172392143,-8.7535724295965,12.9091426524948));
#15185=CARTESIAN_POINT('Ctrl Pts',(3.95807743820715,-5.80714485919301,12.236639786787));
#15186=CARTESIAN_POINT('Ctrl Pts',(4.17236315249286,-3.4442934046707,10.3523286299233));
#15187=CARTESIAN_POINT('Ctrl Pts',(4.38664886677858,-1.08144195014837,8.46801747305969));
#15188=CARTESIAN_POINT('Ctrl Pts',(4.60093458106429,0.229841679453252,5.74510895921686));
#15189=CARTESIAN_POINT('Ctrl Pts',(4.81522029535,1.5411253090549,3.02220044537404));
#15190=CARTESIAN_POINT('Ctrl Pts',(5.02950600963572,1.5411253090549,0.));
#15191=CARTESIAN_POINT('Ctrl Pts',(5.24379172392143,1.5411253090549,-3.02220044537404));
#15192=CARTESIAN_POINT('Ctrl Pts',(5.45807743820715,0.229841679453252,-5.74510895921687));
#15193=CARTESIAN_POINT('Ctrl Pts',(5.67236315249286,-1.08144195014837,-8.4680174730597));
#15194=CARTESIAN_POINT('Ctrl Pts',(5.88664886677858,-3.4442934046707,-10.3523286299233));
#15195=CARTESIAN_POINT('Ctrl Pts',(6.10093458106429,-5.80714485919301,-12.236639786787));
#15196=CARTESIAN_POINT('Ctrl Pts',(6.31522029535001,-8.75357242959651,-12.9091426524948));
#15197=CARTESIAN_POINT('Ctrl Pts',(6.52950600963572,-11.7,-13.5816455182026));
#15198=CARTESIAN_POINT('Ctrl Pts',(6.74379172392144,-14.6464275704035,-12.9091426524948));
#15199=CARTESIAN_POINT('Ctrl Pts',(6.95807743820715,-17.592855140807,-12.236639786787));
#15200=CARTESIAN_POINT('Ctrl Pts',(7.17236315249286,-19.9557065953293,-10.3523286299233));
#15201=CARTESIAN_POINT('Ctrl Pts',(7.38664886677858,-22.3185580498516,-8.4680174730597));
#15202=CARTESIAN_POINT('Ctrl Pts',(7.60093458106429,-23.6298416794532,-5.74510895921687));
#15203=CARTESIAN_POINT('Ctrl Pts',(7.81522029535,-24.9411253090549,-3.02220044537404));
#15204=CARTESIAN_POINT('Ctrl Pts',(8.02950600963572,-24.9411253090549,-6.93889390390723E-15));
#15205=CARTESIAN_POINT('Ctrl Pts',(8.24379172392143,-24.9411253090549,3.02220044537402));
#15206=CARTESIAN_POINT('Ctrl Pts',(8.45807743820715,-23.6298416794532,5.74510895921685));
#15207=CARTESIAN_POINT('Ctrl Pts',(8.67236315249286,-22.3185580498516,8.4680174730597));
#15208=CARTESIAN_POINT('Ctrl Pts',(8.88664886677858,-19.9557065953293,10.3523286299233));
#15209=CARTESIAN_POINT('Ctrl Pts',(9.10093458106429,-17.592855140807,12.236639786787));
#15210=CARTESIAN_POINT('Ctrl Pts',(9.31522029535001,-14.6464275704035,12.9091426524948));
#15211=CARTESIAN_POINT('Ctrl Pts',(9.52950600963572,-11.7,13.5816455182026));
#15212=CARTESIAN_POINT('Ctrl Pts',(9.74379172392144,-8.75357242959651,12.9091426524948));
#15213=CARTESIAN_POINT('Ctrl Pts',(9.95807743820714,-5.80714485919302,12.236639786787));
#15214=CARTESIAN_POINT('Ctrl Pts',(10.1723631524929,-3.4442934046707,10.3523286299233));
#15215=CARTESIAN_POINT('Ctrl Pts',(10.3866488667786,-1.08144195014837,8.4680174730597));
#15216=CARTESIAN_POINT('Ctrl Pts',(10.6009345810643,0.229841679453252,5.74510895921686));
#15217=CARTESIAN_POINT('Ctrl Pts',(10.81522029535,1.5411253090549,3.02220044537402));
#15218=CARTESIAN_POINT('Ctrl Pts',(11.0295060096357,1.5411253090549,6.93889390390723E-15));
#15219=CARTESIAN_POINT('Ctrl Pts',(11.2437917239214,1.54112530905489,-3.02220044537404));
#15220=CARTESIAN_POINT('Ctrl Pts',(11.4580774382071,0.229841679453259,-5.74510895921686));
#15221=CARTESIAN_POINT('Ctrl Pts',(11.6723631524929,-1.08144195014837,-8.4680174730597));
#15222=CARTESIAN_POINT('Ctrl Pts',(11.8866488667786,-3.4442934046707,-10.3523286299233));
#15223=CARTESIAN_POINT('Ctrl Pts',(12.1009345810643,-5.80714485919302,-12.236639786787));
#15224=CARTESIAN_POINT('Ctrl Pts',(12.31522029535,-8.75357242959649,-12.9091426524948));
#15225=CARTESIAN_POINT('Ctrl Pts',(12.5295060096357,-11.7,-13.5816455182026));
#15226=CARTESIAN_POINT('Ctrl Pts',(12.7437917239214,-14.6464275704035,-12.9091426524948));
#15227=CARTESIAN_POINT('Ctrl Pts',(12.9580774382072,-17.592855140807,-12.236639786787));
#15228=CARTESIAN_POINT('Ctrl Pts',(13.1723631524929,-19.9557065953293,-10.3523286299233));
#15229=CARTESIAN_POINT('Ctrl Pts',(13.3866488667786,-22.3185580498516,-8.4680174730597));
#15230=CARTESIAN_POINT('Ctrl Pts',(13.6009345810643,-23.6298416794532,-5.74510895921687));
#15231=CARTESIAN_POINT('Ctrl Pts',(13.81522029535,-24.9411253090549,-3.02220044537403));
#15232=CARTESIAN_POINT('Ctrl Pts',(14.0295060096357,-24.9411253090549,-6.93889390390723E-15));
#15233=CARTESIAN_POINT('Ctrl Pts',(14.2437917239214,-24.9411253090549,3.02220044537403));
#15234=CARTESIAN_POINT('Ctrl Pts',(14.4580774382072,-23.6298416794532,5.74510895921685));
#15235=CARTESIAN_POINT('Ctrl Pts',(14.6723631524929,-22.3185580498516,8.46801747305969));
#15236=CARTESIAN_POINT('Ctrl Pts',(14.8866488667786,-19.9557065953293,10.3523286299233));
#15237=CARTESIAN_POINT('Ctrl Pts',(15.1009345810643,-17.592855140807,12.236639786787));
#15238=CARTESIAN_POINT('Ctrl Pts',(15.31522029535,-14.6464275704035,12.9091426524948));
#15239=CARTESIAN_POINT('Ctrl Pts',(15.5295060096357,-11.7,13.5816455182026));
#15240=CARTESIAN_POINT('Ctrl Pts',(15.7437917239214,-8.75357242959651,12.9091426524948));
#15241=CARTESIAN_POINT('Ctrl Pts',(15.9580774382071,-5.80714485919302,12.236639786787));
#15242=CARTESIAN_POINT('Ctrl Pts',(16.1723631524929,-3.4442934046707,10.3523286299233));
#15243=CARTESIAN_POINT('Ctrl Pts',(16.3866488667786,-1.08144195014837,8.46801747305969));
#15244=CARTESIAN_POINT('Ctrl Pts',(16.6009345810643,0.229841679453266,5.74510895921686));
#15245=CARTESIAN_POINT('Ctrl Pts',(16.81522029535,1.5411253090549,3.02220044537404));
#15246=CARTESIAN_POINT('Ctrl Pts',(17.0295060096357,1.5411253090549,-2.08166817117217E-14));
#15247=CARTESIAN_POINT('Ctrl Pts',(17.2437917239214,1.5411253090549,-3.02220044537405));
#15248=CARTESIAN_POINT('Ctrl Pts',(17.4580774382072,0.229841679453266,-5.74510895921688));
#15249=CARTESIAN_POINT('Ctrl Pts',(17.6723631524929,-1.08144195014837,-8.46801747305971));
#15250=CARTESIAN_POINT('Ctrl Pts',(17.8866488667786,-3.44429340467071,-10.3523286299233));
#15251=CARTESIAN_POINT('Ctrl Pts',(18.1009345810643,-5.80714485919302,-12.236639786787));
#15252=CARTESIAN_POINT('Ctrl Pts',(18.31522029535,-8.75357242959651,-12.9091426524948));
#15253=CARTESIAN_POINT('Ctrl Pts',(18.5295060096357,-11.7,-13.5816455182026));
#15254=CARTESIAN_POINT('Ctrl Pts',(18.7437917239214,-14.6464275704035,-12.9091426524948));
#15255=CARTESIAN_POINT('Ctrl Pts',(18.9580774382071,-17.592855140807,-12.236639786787));
#15256=CARTESIAN_POINT('Ctrl Pts',(19.1723631524929,-19.9557065953293,-10.3523286299233));
#15257=CARTESIAN_POINT('Ctrl Pts',(19.3866488667786,-22.3185580498516,-8.4680174730597));
#15258=CARTESIAN_POINT('Ctrl Pts',(19.6009345810643,-23.6298416794532,-5.74510895921687));
#15259=CARTESIAN_POINT('Ctrl Pts',(19.81522029535,-24.9411253090549,-3.02220044537404));
#15260=CARTESIAN_POINT('Ctrl Pts',(20.0295060096357,-24.9411253090549,0.));
#15261=CARTESIAN_POINT('Ctrl Pts',(20.2437917239214,-24.9411253090549,3.02220044537403));
#15262=CARTESIAN_POINT('Ctrl Pts',(20.4580774382071,-23.6298416794532,5.74510895921685));
#15263=CARTESIAN_POINT('Ctrl Pts',(20.6723631524929,-22.3185580498516,8.46801747305969));
#15264=CARTESIAN_POINT('Ctrl Pts',(20.8866488667786,-19.9557065953293,10.3523286299233));
#15265=CARTESIAN_POINT('Ctrl Pts',(21.1009345810643,-17.5928551408069,12.236639786787));
#15266=CARTESIAN_POINT('Ctrl Pts',(21.31522029535,-14.6464275704035,12.9091426524948));
#15267=CARTESIAN_POINT('Ctrl Pts',(21.5295060096357,-11.7,13.5816455182026));
#15268=CARTESIAN_POINT('Ctrl Pts',(21.7437917239214,-8.75357242959651,12.9091426524948));
#15269=CARTESIAN_POINT('Ctrl Pts',(21.9580774382071,-5.80714485919301,12.236639786787));
#15270=CARTESIAN_POINT('Ctrl Pts',(22.1723631524929,-3.4442934046707,10.3523286299233));
#15271=CARTESIAN_POINT('Ctrl Pts',(22.3866488667786,-1.08144195014837,8.4680174730597));
#15272=CARTESIAN_POINT('Ctrl Pts',(22.6009345810643,0.229841679453259,5.74510895921686));
#15273=CARTESIAN_POINT('Ctrl Pts',(22.81522029535,1.54112530905491,3.02220044537404));
#15274=CARTESIAN_POINT('Ctrl Pts',(23.0295060096357,1.5411253090549,0.));
#15275=CARTESIAN_POINT('Ctrl Pts',(0.970493990364278,1.5411253090549,-1.38777878078145E-14));
#15276=CARTESIAN_POINT('Ctrl Pts',(1.18477970464999,1.54112530905491,-3.02220044537403));
#15277=CARTESIAN_POINT('Ctrl Pts',(1.39906541893571,0.229841679453259,-5.74510895921686));
#15278=CARTESIAN_POINT('Ctrl Pts',(1.61335113322142,-1.08144195014838,-8.4680174730597));
#15279=CARTESIAN_POINT('Ctrl Pts',(1.82763684750713,-3.44429340467071,-10.3523286299233));
#15280=CARTESIAN_POINT('Ctrl Pts',(2.04192256179285,-5.80714485919301,-12.236639786787));
#15281=CARTESIAN_POINT('Ctrl Pts',(2.25620827607856,-8.75357242959651,-12.9091426524948));
#15282=CARTESIAN_POINT('Ctrl Pts',(2.47049399036428,-11.7,-13.5816455182026));
#15283=CARTESIAN_POINT('Ctrl Pts',(2.68477970464999,-14.6464275704035,-12.9091426524948));
#15284=CARTESIAN_POINT('Ctrl Pts',(2.89906541893571,-17.592855140807,-12.236639786787));
#15285=CARTESIAN_POINT('Ctrl Pts',(3.11335113322142,-19.9557065953293,-10.3523286299233));
#15286=CARTESIAN_POINT('Ctrl Pts',(3.32763684750713,-22.3185580498516,-8.4680174730597));
#15287=CARTESIAN_POINT('Ctrl Pts',(3.54192256179285,-23.6298416794532,-5.74510895921686));
#15288=CARTESIAN_POINT('Ctrl Pts',(3.75620827607856,-24.9411253090549,-3.02220044537403));
#15289=CARTESIAN_POINT('Ctrl Pts',(3.97049399036428,-24.9411253090549,3.46944695195361E-15));
#15290=CARTESIAN_POINT('Ctrl Pts',(4.18477970464999,-24.9411253090549,3.02220044537403));
#15291=CARTESIAN_POINT('Ctrl Pts',(4.39906541893571,-23.6298416794532,5.74510895921686));
#15292=CARTESIAN_POINT('Ctrl Pts',(4.61335113322142,-22.3185580498516,8.46801747305969));
#15293=CARTESIAN_POINT('Ctrl Pts',(4.82763684750714,-19.9557065953293,10.3523286299233));
#15294=CARTESIAN_POINT('Ctrl Pts',(5.04192256179285,-17.592855140807,12.2366397867869));
#15295=CARTESIAN_POINT('Ctrl Pts',(5.25620827607856,-14.6464275704035,12.9091426524948));
#15296=CARTESIAN_POINT('Ctrl Pts',(5.47049399036428,-11.7,13.5816455182026));
#15297=CARTESIAN_POINT('Ctrl Pts',(5.68477970464999,-8.75357242959651,12.9091426524948));
#15298=CARTESIAN_POINT('Ctrl Pts',(5.89906541893571,-5.80714485919302,12.236639786787));
#15299=CARTESIAN_POINT('Ctrl Pts',(6.11335113322142,-3.4442934046707,10.3523286299233));
#15300=CARTESIAN_POINT('Ctrl Pts',(6.32763684750713,-1.08144195014838,8.4680174730597));
#15301=CARTESIAN_POINT('Ctrl Pts',(6.54192256179285,0.229841679453252,5.74510895921686));
#15302=CARTESIAN_POINT('Ctrl Pts',(6.75620827607856,1.5411253090549,3.02220044537404));
#15303=CARTESIAN_POINT('Ctrl Pts',(6.97049399036428,1.5411253090549,-1.38777878078145E-14));
#15304=CARTESIAN_POINT('Ctrl Pts',(7.18477970464999,1.5411253090549,-3.02220044537404));
#15305=CARTESIAN_POINT('Ctrl Pts',(7.39906541893571,0.229841679453259,-5.74510895921689));
#15306=CARTESIAN_POINT('Ctrl Pts',(7.61335113322142,-1.08144195014838,-8.46801747305971));
#15307=CARTESIAN_POINT('Ctrl Pts',(7.82763684750713,-3.4442934046707,-10.3523286299233));
#15308=CARTESIAN_POINT('Ctrl Pts',(8.04192256179285,-5.80714485919302,-12.236639786787));
#15309=CARTESIAN_POINT('Ctrl Pts',(8.25620827607856,-8.75357242959651,-12.9091426524948));
#15310=CARTESIAN_POINT('Ctrl Pts',(8.47049399036428,-11.7,-13.5816455182026));
#15311=CARTESIAN_POINT('Ctrl Pts',(8.68477970464999,-14.6464275704035,-12.9091426524948));
#15312=CARTESIAN_POINT('Ctrl Pts',(8.89906541893571,-17.592855140807,-12.236639786787));
#15313=CARTESIAN_POINT('Ctrl Pts',(9.11335113322142,-19.9557065953293,-10.3523286299233));
#15314=CARTESIAN_POINT('Ctrl Pts',(9.32763684750714,-22.3185580498516,-8.4680174730597));
#15315=CARTESIAN_POINT('Ctrl Pts',(9.54192256179285,-23.6298416794532,-5.74510895921687));
#15316=CARTESIAN_POINT('Ctrl Pts',(9.75620827607856,-24.9411253090549,-3.02220044537404));
#15317=CARTESIAN_POINT('Ctrl Pts',(9.97049399036428,-24.9411253090549,-6.93889390390723E-15));
#15318=CARTESIAN_POINT('Ctrl Pts',(10.18477970465,-24.9411253090549,3.02220044537403));
#15319=CARTESIAN_POINT('Ctrl Pts',(10.3990654189357,-23.6298416794532,5.74510895921686));
#15320=CARTESIAN_POINT('Ctrl Pts',(10.6133511332214,-22.3185580498516,8.4680174730597));
#15321=CARTESIAN_POINT('Ctrl Pts',(10.8276368475071,-19.9557065953293,10.3523286299233));
#15322=CARTESIAN_POINT('Ctrl Pts',(11.0419225617928,-17.592855140807,12.236639786787));
#15323=CARTESIAN_POINT('Ctrl Pts',(11.2562082760786,-14.6464275704035,12.9091426524948));
#15324=CARTESIAN_POINT('Ctrl Pts',(11.4704939903643,-11.7,13.5816455182026));
#15325=CARTESIAN_POINT('Ctrl Pts',(11.68477970465,-8.75357242959651,12.9091426524948));
#15326=CARTESIAN_POINT('Ctrl Pts',(11.8990654189357,-5.80714485919301,12.236639786787));
#15327=CARTESIAN_POINT('Ctrl Pts',(12.1133511332214,-3.4442934046707,10.3523286299233));
#15328=CARTESIAN_POINT('Ctrl Pts',(12.3276368475071,-1.08144195014836,8.4680174730597));
#15329=CARTESIAN_POINT('Ctrl Pts',(12.5419225617929,0.229841679453266,5.74510895921686));
#15330=CARTESIAN_POINT('Ctrl Pts',(12.7562082760786,1.5411253090549,3.02220044537403));
#15331=CARTESIAN_POINT('Ctrl Pts',(12.9704939903643,1.5411253090549,-2.08166817117217E-14));
#15332=CARTESIAN_POINT('Ctrl Pts',(13.18477970465,1.5411253090549,-3.02220044537405));
#15333=CARTESIAN_POINT('Ctrl Pts',(13.3990654189357,0.229841679453252,-5.74510895921687));
#15334=CARTESIAN_POINT('Ctrl Pts',(13.6133511332214,-1.08144195014838,-8.46801747305971));
#15335=CARTESIAN_POINT('Ctrl Pts',(13.8276368475071,-3.44429340467069,-10.3523286299233));
#15336=CARTESIAN_POINT('Ctrl Pts',(14.0419225617929,-5.80714485919301,-12.236639786787));
#15337=CARTESIAN_POINT('Ctrl Pts',(14.2562082760786,-8.75357242959651,-12.9091426524948));
#15338=CARTESIAN_POINT('Ctrl Pts',(14.4704939903643,-11.7,-13.5816455182026));
#15339=CARTESIAN_POINT('Ctrl Pts',(14.68477970465,-14.6464275704035,-12.9091426524948));
#15340=CARTESIAN_POINT('Ctrl Pts',(14.8990654189357,-17.592855140807,-12.236639786787));
#15341=CARTESIAN_POINT('Ctrl Pts',(15.1133511332214,-19.9557065953293,-10.3523286299233));
#15342=CARTESIAN_POINT('Ctrl Pts',(15.3276368475071,-22.3185580498516,-8.46801747305969));
#15343=CARTESIAN_POINT('Ctrl Pts',(15.5419225617929,-23.6298416794532,-5.74510895921687));
#15344=CARTESIAN_POINT('Ctrl Pts',(15.7562082760786,-24.9411253090549,-3.02220044537403));
#15345=CARTESIAN_POINT('Ctrl Pts',(15.9704939903643,-24.9411253090549,-6.93889390390723E-15));
#15346=CARTESIAN_POINT('Ctrl Pts',(16.18477970465,-24.9411253090549,3.02220044537403));
#15347=CARTESIAN_POINT('Ctrl Pts',(16.3990654189357,-23.6298416794532,5.74510895921686));
#15348=CARTESIAN_POINT('Ctrl Pts',(16.6133511332214,-22.3185580498516,8.46801747305969));
#15349=CARTESIAN_POINT('Ctrl Pts',(16.8276368475071,-19.9557065953293,10.3523286299233));
#15350=CARTESIAN_POINT('Ctrl Pts',(17.0419225617928,-17.592855140807,12.236639786787));
#15351=CARTESIAN_POINT('Ctrl Pts',(17.2562082760786,-14.6464275704035,12.9091426524948));
#15352=CARTESIAN_POINT('Ctrl Pts',(17.4704939903643,-11.7,13.5816455182026));
#15353=CARTESIAN_POINT('Ctrl Pts',(17.68477970465,-8.75357242959651,12.9091426524948));
#15354=CARTESIAN_POINT('Ctrl Pts',(17.8990654189357,-5.80714485919301,12.236639786787));
#15355=CARTESIAN_POINT('Ctrl Pts',(18.1133511332214,-3.4442934046707,10.3523286299233));
#15356=CARTESIAN_POINT('Ctrl Pts',(18.3276368475071,-1.08144195014837,8.46801747305969));
#15357=CARTESIAN_POINT('Ctrl Pts',(18.5419225617928,0.229841679453252,5.74510895921686));
#15358=CARTESIAN_POINT('Ctrl Pts',(18.7562082760786,1.5411253090549,3.02220044537405));
#15359=CARTESIAN_POINT('Ctrl Pts',(18.9704939903643,1.5411253090549,-1.38777878078145E-14));
#15360=CARTESIAN_POINT('Ctrl Pts',(19.18477970465,1.5411253090549,-3.02220044537404));
#15361=CARTESIAN_POINT('Ctrl Pts',(19.3990654189357,0.229841679453259,-5.74510895921686));
#15362=CARTESIAN_POINT('Ctrl Pts',(19.6133511332214,-1.08144195014838,-8.4680174730597));
#15363=CARTESIAN_POINT('Ctrl Pts',(19.8276368475071,-3.4442934046707,-10.3523286299233));
#15364=CARTESIAN_POINT('Ctrl Pts',(20.0419225617929,-5.80714485919302,-12.236639786787));
#15365=CARTESIAN_POINT('Ctrl Pts',(20.2562082760786,-8.75357242959651,-12.9091426524948));
#15366=CARTESIAN_POINT('Ctrl Pts',(20.4704939903643,-11.7,-13.5816455182026));
#15367=CARTESIAN_POINT('Ctrl Pts',(20.68477970465,-14.6464275704035,-12.9091426524948));
#15368=CARTESIAN_POINT('Ctrl Pts',(20.8990654189357,-17.592855140807,-12.236639786787));
#15369=CARTESIAN_POINT('Ctrl Pts',(21.1133511332214,-19.9557065953293,-10.3523286299233));
#15370=CARTESIAN_POINT('Ctrl Pts',(21.3276368475071,-22.3185580498516,-8.4680174730597));
#15371=CARTESIAN_POINT('Ctrl Pts',(21.5419225617929,-23.6298416794532,-5.74510895921687));
#15372=CARTESIAN_POINT('Ctrl Pts',(21.7562082760786,-24.9411253090549,-3.02220044537404));
#15373=CARTESIAN_POINT('Ctrl Pts',(21.9704939903643,-24.9411253090549,-3.46944695195361E-15));
#15374=CARTESIAN_POINT('Ctrl Pts',(22.18477970465,-24.9411253090549,3.02220044537403));
#15375=CARTESIAN_POINT('Ctrl Pts',(22.3990654189357,-23.6298416794532,5.74510895921686));
#15376=CARTESIAN_POINT('Ctrl Pts',(22.6133511332214,-22.3185580498516,8.46801747305969));
#15377=CARTESIAN_POINT('Ctrl Pts',(22.8276368475071,-19.9557065953293,10.3523286299233));
#15378=CARTESIAN_POINT('Ctrl Pts',(23.0419225617928,-17.592855140807,12.236639786787));
#15379=CARTESIAN_POINT('Ctrl Pts',(23.2562082760786,-14.6464275704035,12.9091426524948));
#15380=CARTESIAN_POINT('Ctrl Pts',(23.4704939903643,-11.7,13.5816455182026));
#15381=CARTESIAN_POINT('Ctrl Pts',(23.68477970465,-8.75357242959651,12.9091426524948));
#15382=CARTESIAN_POINT('Ctrl Pts',(23.8990654189357,-5.80714485919302,12.236639786787));
#15383=CARTESIAN_POINT('Ctrl Pts',(24.1133511332214,-3.4442934046707,10.3523286299233));
#15384=CARTESIAN_POINT('Ctrl Pts',(24.3276368475071,-1.08144195014837,8.46801747305969));
#15385=CARTESIAN_POINT('Ctrl Pts',(24.5419225617928,0.229841679453252,5.74510895921686));
#15386=CARTESIAN_POINT('Ctrl Pts',(24.7562082760786,1.5411253090549,3.02220044537404));
#15387=CARTESIAN_POINT('Ctrl Pts',(24.9704939903643,1.5411253090549,0.));
#15388=CARTESIAN_POINT('Ctrl Pts',(0.654743522119005,2.81197461594778,-1.40439689870177E-14));
#15389=CARTESIAN_POINT('Ctrl Pts',(0.869029236404722,2.81197461594777,-3.31226350660561));
#15390=CARTESIAN_POINT('Ctrl Pts',(1.08331495069043,1.37483734075911,-6.2965098083465));
#15391=CARTESIAN_POINT('Ctrl Pts',(1.29760066497615,-0.0622999344295592,
-9.28075611008744));
#15392=CARTESIAN_POINT('Ctrl Pts',(1.51188637926186,-2.65193182212374,-11.3459186275249));
#15393=CARTESIAN_POINT('Ctrl Pts',(1.72617209354758,-5.24156370981795,-13.4110811449623));
#15394=CARTESIAN_POINT('Ctrl Pts',(1.94045780783329,-8.47078185490896,-14.1481291139616));
#15395=CARTESIAN_POINT('Ctrl Pts',(2.15474352211901,-11.7,-14.8851770829609));
#15396=CARTESIAN_POINT('Ctrl Pts',(2.36902923640472,-14.929218145091,-14.1481291139616));
#15397=CARTESIAN_POINT('Ctrl Pts',(2.58331495069044,-18.158436290182,-13.4110811449623));
#15398=CARTESIAN_POINT('Ctrl Pts',(2.79760066497615,-20.7480681778762,-11.3459186275249));
#15399=CARTESIAN_POINT('Ctrl Pts',(3.01188637926186,-23.3377000655704,-9.28075611008745));
#15400=CARTESIAN_POINT('Ctrl Pts',(3.22617209354758,-24.7748373407591,-6.29650980834652));
#15401=CARTESIAN_POINT('Ctrl Pts',(3.44045780783329,-26.2119746159478,-3.31226350660559));
#15402=CARTESIAN_POINT('Ctrl Pts',(3.65474352211901,-26.2119746159477,0.));
#15403=CARTESIAN_POINT('Ctrl Pts',(3.86902923640472,-26.2119746159478,3.31226350660556));
#15404=CARTESIAN_POINT('Ctrl Pts',(4.08331495069043,-24.7748373407591,6.2965098083465));
#15405=CARTESIAN_POINT('Ctrl Pts',(4.29760066497615,-23.3377000655704,9.28075611008741));
#15406=CARTESIAN_POINT('Ctrl Pts',(4.51188637926187,-20.7480681778762,11.3459186275248));
#15407=CARTESIAN_POINT('Ctrl Pts',(4.72617209354758,-18.158436290182,13.4110811449623));
#15408=CARTESIAN_POINT('Ctrl Pts',(4.94045780783329,-14.929218145091,14.1481291139616));
#15409=CARTESIAN_POINT('Ctrl Pts',(5.15474352211901,-11.7,14.8851770829609));
#15410=CARTESIAN_POINT('Ctrl Pts',(5.36902923640472,-8.47078185490897,14.1481291139616));
#15411=CARTESIAN_POINT('Ctrl Pts',(5.58331495069043,-5.24156370981795,13.4110811449623));
#15412=CARTESIAN_POINT('Ctrl Pts',(5.79760066497615,-2.65193182212374,11.3459186275248));
#15413=CARTESIAN_POINT('Ctrl Pts',(6.01188637926187,-0.0622999344295592,
9.28075611008741));
#15414=CARTESIAN_POINT('Ctrl Pts',(6.22617209354758,1.3748373407591,6.2965098083465));
#15415=CARTESIAN_POINT('Ctrl Pts',(6.44045780783329,2.81197461594777,3.31226350660556));
#15416=CARTESIAN_POINT('Ctrl Pts',(6.65474352211901,2.81197461594778,-2.10659534805265E-14));
#15417=CARTESIAN_POINT('Ctrl Pts',(6.86902923640472,2.81197461594777,-3.31226350660559));
#15418=CARTESIAN_POINT('Ctrl Pts',(7.08331495069044,1.37483734075912,-6.29650980834652));
#15419=CARTESIAN_POINT('Ctrl Pts',(7.29760066497615,-0.0622999344295448,
-9.28075611008746));
#15420=CARTESIAN_POINT('Ctrl Pts',(7.51188637926187,-2.65193182212374,-11.3459186275249));
#15421=CARTESIAN_POINT('Ctrl Pts',(7.72617209354758,-5.24156370981795,-13.4110811449623));
#15422=CARTESIAN_POINT('Ctrl Pts',(7.9404578078333,-8.47078185490895,-14.1481291139616));
#15423=CARTESIAN_POINT('Ctrl Pts',(8.15474352211901,-11.7,-14.8851770829609));
#15424=CARTESIAN_POINT('Ctrl Pts',(8.36902923640472,-14.929218145091,-14.1481291139616));
#15425=CARTESIAN_POINT('Ctrl Pts',(8.58331495069044,-18.158436290182,-13.4110811449623));
#15426=CARTESIAN_POINT('Ctrl Pts',(8.79760066497615,-20.7480681778762,-11.3459186275249));
#15427=CARTESIAN_POINT('Ctrl Pts',(9.01188637926186,-23.3377000655704,-9.28075611008744));
#15428=CARTESIAN_POINT('Ctrl Pts',(9.22617209354758,-24.7748373407591,-6.29650980834652));
#15429=CARTESIAN_POINT('Ctrl Pts',(9.44045780783329,-26.2119746159478,-3.3122635066056));
#15430=CARTESIAN_POINT('Ctrl Pts',(9.65474352211901,-26.2119746159477,-1.40439689870177E-14));
#15431=CARTESIAN_POINT('Ctrl Pts',(9.86902923640472,-26.2119746159478,3.31226350660556));
#15432=CARTESIAN_POINT('Ctrl Pts',(10.0833149506904,-24.7748373407591,6.29650980834649));
#15433=CARTESIAN_POINT('Ctrl Pts',(10.2976006649762,-23.3377000655704,9.28075611008742));
#15434=CARTESIAN_POINT('Ctrl Pts',(10.5118863792619,-20.7480681778762,11.3459186275248));
#15435=CARTESIAN_POINT('Ctrl Pts',(10.7261720935476,-18.158436290182,13.4110811449623));
#15436=CARTESIAN_POINT('Ctrl Pts',(10.9404578078333,-14.929218145091,14.1481291139616));
#15437=CARTESIAN_POINT('Ctrl Pts',(11.154743522119,-11.7,14.8851770829608));
#15438=CARTESIAN_POINT('Ctrl Pts',(11.3690292364047,-8.47078185490896,14.1481291139616));
#15439=CARTESIAN_POINT('Ctrl Pts',(11.5833149506904,-5.24156370981795,13.4110811449623));
#15440=CARTESIAN_POINT('Ctrl Pts',(11.7976006649762,-2.65193182212374,11.3459186275248));
#15441=CARTESIAN_POINT('Ctrl Pts',(12.0118863792619,-0.0622999344295592,
9.28075611008742));
#15442=CARTESIAN_POINT('Ctrl Pts',(12.2261720935476,1.3748373407591,6.29650980834649));
#15443=CARTESIAN_POINT('Ctrl Pts',(12.4404578078333,2.81197461594777,3.31226350660557));
#15444=CARTESIAN_POINT('Ctrl Pts',(12.654743522119,2.81197461594777,0.));
#15445=CARTESIAN_POINT('Ctrl Pts',(12.8690292364047,2.81197461594777,-3.31226350660558));
#15446=CARTESIAN_POINT('Ctrl Pts',(13.0833149506904,1.37483734075912,-6.29650980834652));
#15447=CARTESIAN_POINT('Ctrl Pts',(13.2976006649762,-0.0622999344295448,
-9.28075611008746));
#15448=CARTESIAN_POINT('Ctrl Pts',(13.5118863792619,-2.65193182212374,-11.3459186275249));
#15449=CARTESIAN_POINT('Ctrl Pts',(13.7261720935476,-5.24156370981795,-13.4110811449623));
#15450=CARTESIAN_POINT('Ctrl Pts',(13.9404578078333,-8.47078185490895,-14.1481291139616));
#15451=CARTESIAN_POINT('Ctrl Pts',(14.154743522119,-11.7,-14.8851770829609));
#15452=CARTESIAN_POINT('Ctrl Pts',(14.3690292364047,-14.929218145091,-14.1481291139616));
#15453=CARTESIAN_POINT('Ctrl Pts',(14.5833149506904,-18.158436290182,-13.4110811449623));
#15454=CARTESIAN_POINT('Ctrl Pts',(14.7976006649761,-20.7480681778762,-11.3459186275249));
#15455=CARTESIAN_POINT('Ctrl Pts',(15.0118863792619,-23.3377000655704,-9.28075611008744));
#15456=CARTESIAN_POINT('Ctrl Pts',(15.2261720935476,-24.7748373407591,-6.29650980834651));
#15457=CARTESIAN_POINT('Ctrl Pts',(15.4404578078333,-26.2119746159478,-3.31226350660559));
#15458=CARTESIAN_POINT('Ctrl Pts',(15.654743522119,-26.2119746159478,-1.40439689870177E-14));
#15459=CARTESIAN_POINT('Ctrl Pts',(15.8690292364047,-26.2119746159478,3.31226350660556));
#15460=CARTESIAN_POINT('Ctrl Pts',(16.0833149506904,-24.7748373407591,6.29650980834649));
#15461=CARTESIAN_POINT('Ctrl Pts',(16.2976006649761,-23.3377000655704,9.28075611008742));
#15462=CARTESIAN_POINT('Ctrl Pts',(16.5118863792619,-20.7480681778762,11.3459186275248));
#15463=CARTESIAN_POINT('Ctrl Pts',(16.7261720935476,-18.158436290182,13.4110811449623));
#15464=CARTESIAN_POINT('Ctrl Pts',(16.9404578078333,-14.929218145091,14.1481291139616));
#15465=CARTESIAN_POINT('Ctrl Pts',(17.154743522119,-11.7,14.8851770829609));
#15466=CARTESIAN_POINT('Ctrl Pts',(17.3690292364047,-8.47078185490896,14.1481291139616));
#15467=CARTESIAN_POINT('Ctrl Pts',(17.5833149506904,-5.24156370981795,13.4110811449623));
#15468=CARTESIAN_POINT('Ctrl Pts',(17.7976006649762,-2.65193182212374,11.3459186275248));
#15469=CARTESIAN_POINT('Ctrl Pts',(18.0118863792619,-0.0622999344295592,
9.28075611008742));
#15470=CARTESIAN_POINT('Ctrl Pts',(18.2261720935476,1.37483734075912,6.29650980834649));
#15471=CARTESIAN_POINT('Ctrl Pts',(18.4404578078333,2.81197461594777,3.31226350660556));
#15472=CARTESIAN_POINT('Ctrl Pts',(18.654743522119,2.81197461594778,0.));
#15473=CARTESIAN_POINT('Ctrl Pts',(18.8690292364047,2.81197461594775,-3.31226350660559));
#15474=CARTESIAN_POINT('Ctrl Pts',(19.0833149506904,1.37483734075912,-6.29650980834651));
#15475=CARTESIAN_POINT('Ctrl Pts',(19.2976006649762,-0.0622999344295592,
-9.28075611008743));
#15476=CARTESIAN_POINT('Ctrl Pts',(19.5118863792619,-2.65193182212375,-11.3459186275249));
#15477=CARTESIAN_POINT('Ctrl Pts',(19.7261720935476,-5.24156370981795,-13.4110811449623));
#15478=CARTESIAN_POINT('Ctrl Pts',(19.9404578078333,-8.47078185490895,-14.1481291139616));
#15479=CARTESIAN_POINT('Ctrl Pts',(20.154743522119,-11.7,-14.8851770829609));
#15480=CARTESIAN_POINT('Ctrl Pts',(20.3690292364047,-14.929218145091,-14.1481291139616));
#15481=CARTESIAN_POINT('Ctrl Pts',(20.5833149506904,-18.158436290182,-13.4110811449623));
#15482=CARTESIAN_POINT('Ctrl Pts',(20.7976006649762,-20.7480681778762,-11.3459186275249));
#15483=CARTESIAN_POINT('Ctrl Pts',(21.0118863792619,-23.3377000655704,-9.28075611008745));
#15484=CARTESIAN_POINT('Ctrl Pts',(21.2261720935476,-24.7748373407591,-6.29650980834651));
#15485=CARTESIAN_POINT('Ctrl Pts',(21.4404578078333,-26.2119746159478,-3.3122635066056));
#15486=CARTESIAN_POINT('Ctrl Pts',(21.654743522119,-26.2119746159478,-1.75549612337721E-14));
#15487=CARTESIAN_POINT('Ctrl Pts',(21.8690292364047,-26.2119746159478,3.31226350660556));
#15488=CARTESIAN_POINT('Ctrl Pts',(22.0833149506904,-24.7748373407591,6.2965098083465));
#15489=CARTESIAN_POINT('Ctrl Pts',(22.2976006649761,-23.3377000655704,9.28075611008742));
#15490=CARTESIAN_POINT('Ctrl Pts',(22.5118863792619,-20.7480681778762,11.3459186275248));
#15491=CARTESIAN_POINT('Ctrl Pts',(22.7261720935476,-18.158436290182,13.4110811449623));
#15492=CARTESIAN_POINT('Ctrl Pts',(22.9404578078333,-14.929218145091,14.1481291139616));
#15493=CARTESIAN_POINT('Ctrl Pts',(23.154743522119,-11.7,14.8851770829608));
#15494=CARTESIAN_POINT('Ctrl Pts',(23.3690292364047,-8.47078185490898,14.1481291139616));
#15495=CARTESIAN_POINT('Ctrl Pts',(23.5833149506904,-5.24156370981795,13.4110811449623));
#15496=CARTESIAN_POINT('Ctrl Pts',(23.7976006649762,-2.65193182212374,11.3459186275248));
#15497=CARTESIAN_POINT('Ctrl Pts',(24.0118863792619,-0.0622999344295592,
9.28075611008742));
#15498=CARTESIAN_POINT('Ctrl Pts',(24.2261720935476,1.37483734075911,6.29650980834651));
#15499=CARTESIAN_POINT('Ctrl Pts',(24.4404578078333,2.81197461594777,3.31226350660555));
#15500=CARTESIAN_POINT('Ctrl Pts',(24.654743522119,2.81197461594778,-7.02198449350884E-15));
#15501=CARTESIAN_POINT('Ctrl Pts',(-0.65474352211901,2.81197461594778,-2.10659534805265E-14));
#15502=CARTESIAN_POINT('Ctrl Pts',(-0.440457807833293,2.81197461594777,
-3.31226350660559));
#15503=CARTESIAN_POINT('Ctrl Pts',(-0.226172093547581,1.37483734075912,
-6.29650980834653));
#15504=CARTESIAN_POINT('Ctrl Pts',(-0.0118863792618643,-0.0622999344295592,
-9.28075611008746));
#15505=CARTESIAN_POINT('Ctrl Pts',(0.202399335023847,-2.65193182212374,
-11.3459186275249));
#15506=CARTESIAN_POINT('Ctrl Pts',(0.416685049309566,-5.24156370981794,
-13.4110811449623));
#15507=CARTESIAN_POINT('Ctrl Pts',(0.630970763595276,-8.47078185490896,
-14.1481291139616));
#15508=CARTESIAN_POINT('Ctrl Pts',(0.845256477880995,-11.7,-14.8851770829609));
#15509=CARTESIAN_POINT('Ctrl Pts',(1.05954219216671,-14.929218145091,-14.1481291139616));
#15510=CARTESIAN_POINT('Ctrl Pts',(1.27382790645242,-18.158436290182,-13.4110811449623));
#15511=CARTESIAN_POINT('Ctrl Pts',(1.48811362073813,-20.7480681778762,-11.3459186275249));
#15512=CARTESIAN_POINT('Ctrl Pts',(1.70239933502385,-23.3377000655704,-9.28075611008745));
#15513=CARTESIAN_POINT('Ctrl Pts',(1.91668504930956,-24.7748373407591,-6.29650980834651));
#15514=CARTESIAN_POINT('Ctrl Pts',(2.13097076359528,-26.2119746159478,-3.31226350660559));
#15515=CARTESIAN_POINT('Ctrl Pts',(2.34525647788099,-26.2119746159477,-1.05329767402633E-14));
#15516=CARTESIAN_POINT('Ctrl Pts',(2.55954219216671,-26.2119746159478,3.31226350660556));
#15517=CARTESIAN_POINT('Ctrl Pts',(2.77382790645242,-24.7748373407591,6.29650980834649));
#15518=CARTESIAN_POINT('Ctrl Pts',(2.98811362073814,-23.3377000655704,9.28075611008741));
#15519=CARTESIAN_POINT('Ctrl Pts',(3.20239933502385,-20.7480681778762,11.3459186275248));
#15520=CARTESIAN_POINT('Ctrl Pts',(3.41668504930956,-18.158436290182,13.4110811449623));
#15521=CARTESIAN_POINT('Ctrl Pts',(3.63097076359528,-14.929218145091,14.1481291139616));
#15522=CARTESIAN_POINT('Ctrl Pts',(3.84525647788099,-11.7,14.8851770829609));
#15523=CARTESIAN_POINT('Ctrl Pts',(4.05954219216671,-8.47078185490896,14.1481291139616));
#15524=CARTESIAN_POINT('Ctrl Pts',(4.27382790645242,-5.24156370981795,13.4110811449623));
#15525=CARTESIAN_POINT('Ctrl Pts',(4.48811362073814,-2.65193182212374,11.3459186275248));
#15526=CARTESIAN_POINT('Ctrl Pts',(4.70239933502385,-0.0622999344295592,
9.28075611008741));
#15527=CARTESIAN_POINT('Ctrl Pts',(4.91668504930956,1.37483734075912,6.2965098083465));
#15528=CARTESIAN_POINT('Ctrl Pts',(5.13097076359528,2.81197461594777,3.31226350660557));
#15529=CARTESIAN_POINT('Ctrl Pts',(5.34525647788099,2.81197461594778,0.));
#15530=CARTESIAN_POINT('Ctrl Pts',(5.55954219216671,2.81197461594777,-3.31226350660558));
#15531=CARTESIAN_POINT('Ctrl Pts',(5.77382790645242,1.37483734075912,-6.29650980834652));
#15532=CARTESIAN_POINT('Ctrl Pts',(5.98811362073814,-0.0622999344295592,
-9.28075611008745));
#15533=CARTESIAN_POINT('Ctrl Pts',(6.20239933502385,-2.65193182212375,-11.3459186275249));
#15534=CARTESIAN_POINT('Ctrl Pts',(6.41668504930957,-5.24156370981794,-13.4110811449623));
#15535=CARTESIAN_POINT('Ctrl Pts',(6.63097076359528,-8.47078185490895,-14.1481291139616));
#15536=CARTESIAN_POINT('Ctrl Pts',(6.84525647788099,-11.7,-14.8851770829609));
#15537=CARTESIAN_POINT('Ctrl Pts',(7.05954219216671,-14.929218145091,-14.1481291139616));
#15538=CARTESIAN_POINT('Ctrl Pts',(7.27382790645242,-18.158436290182,-13.4110811449623));
#15539=CARTESIAN_POINT('Ctrl Pts',(7.48811362073814,-20.7480681778762,-11.3459186275249));
#15540=CARTESIAN_POINT('Ctrl Pts',(7.70239933502385,-23.3377000655704,-9.28075611008746));
#15541=CARTESIAN_POINT('Ctrl Pts',(7.91668504930956,-24.7748373407591,-6.29650980834652));
#15542=CARTESIAN_POINT('Ctrl Pts',(8.13097076359528,-26.2119746159478,-3.3122635066056));
#15543=CARTESIAN_POINT('Ctrl Pts',(8.34525647788099,-26.2119746159478,-1.40439689870177E-14));
#15544=CARTESIAN_POINT('Ctrl Pts',(8.55954219216671,-26.2119746159478,3.31226350660556));
#15545=CARTESIAN_POINT('Ctrl Pts',(8.77382790645242,-24.7748373407591,6.29650980834649));
#15546=CARTESIAN_POINT('Ctrl Pts',(8.98811362073814,-23.3377000655704,9.28075611008742));
#15547=CARTESIAN_POINT('Ctrl Pts',(9.20239933502385,-20.7480681778762,11.3459186275248));
#15548=CARTESIAN_POINT('Ctrl Pts',(9.41668504930956,-18.158436290182,13.4110811449623));
#15549=CARTESIAN_POINT('Ctrl Pts',(9.63097076359528,-14.929218145091,14.1481291139616));
#15550=CARTESIAN_POINT('Ctrl Pts',(9.84525647788099,-11.7,14.8851770829608));
#15551=CARTESIAN_POINT('Ctrl Pts',(10.0595421921667,-8.47078185490896,14.1481291139616));
#15552=CARTESIAN_POINT('Ctrl Pts',(10.2738279064524,-5.24156370981795,13.4110811449623));
#15553=CARTESIAN_POINT('Ctrl Pts',(10.4881136207381,-2.65193182212374,11.3459186275248));
#15554=CARTESIAN_POINT('Ctrl Pts',(10.7023993350239,-0.0622999344295592,
9.28075611008741));
#15555=CARTESIAN_POINT('Ctrl Pts',(10.9166850493096,1.37483734075912,6.29650980834649));
#15556=CARTESIAN_POINT('Ctrl Pts',(11.1309707635953,2.81197461594777,3.31226350660557));
#15557=CARTESIAN_POINT('Ctrl Pts',(11.345256477881,2.81197461594777,3.51099224675442E-15));
#15558=CARTESIAN_POINT('Ctrl Pts',(11.5595421921667,2.81197461594777,-3.31226350660558));
#15559=CARTESIAN_POINT('Ctrl Pts',(11.7738279064524,1.37483734075912,-6.29650980834651));
#15560=CARTESIAN_POINT('Ctrl Pts',(11.9881136207381,-0.062299934429552,
-9.28075611008743));
#15561=CARTESIAN_POINT('Ctrl Pts',(12.2023993350239,-2.65193182212375,-11.3459186275249));
#15562=CARTESIAN_POINT('Ctrl Pts',(12.4166850493096,-5.24156370981794,-13.4110811449623));
#15563=CARTESIAN_POINT('Ctrl Pts',(12.6309707635953,-8.47078185490895,-14.1481291139616));
#15564=CARTESIAN_POINT('Ctrl Pts',(12.845256477881,-11.7,-14.8851770829609));
#15565=CARTESIAN_POINT('Ctrl Pts',(13.0595421921667,-14.929218145091,-14.1481291139616));
#15566=CARTESIAN_POINT('Ctrl Pts',(13.2738279064524,-18.158436290182,-13.4110811449623));
#15567=CARTESIAN_POINT('Ctrl Pts',(13.4881136207381,-20.7480681778762,-11.3459186275249));
#15568=CARTESIAN_POINT('Ctrl Pts',(13.7023993350239,-23.3377000655704,-9.28075611008744));
#15569=CARTESIAN_POINT('Ctrl Pts',(13.9166850493096,-24.7748373407591,-6.29650980834652));
#15570=CARTESIAN_POINT('Ctrl Pts',(14.1309707635953,-26.2119746159478,-3.3122635066056));
#15571=CARTESIAN_POINT('Ctrl Pts',(14.345256477881,-26.2119746159477,-7.02198449350884E-15));
#15572=CARTESIAN_POINT('Ctrl Pts',(14.5595421921667,-26.2119746159478,3.31226350660556));
#15573=CARTESIAN_POINT('Ctrl Pts',(14.7738279064524,-24.7748373407591,6.29650980834649));
#15574=CARTESIAN_POINT('Ctrl Pts',(14.9881136207381,-23.3377000655704,9.28075611008741));
#15575=CARTESIAN_POINT('Ctrl Pts',(15.2023993350239,-20.7480681778762,11.3459186275248));
#15576=CARTESIAN_POINT('Ctrl Pts',(15.4166850493096,-18.158436290182,13.4110811449623));
#15577=CARTESIAN_POINT('Ctrl Pts',(15.6309707635953,-14.929218145091,14.1481291139616));
#15578=CARTESIAN_POINT('Ctrl Pts',(15.845256477881,-11.7,14.8851770829609));
#15579=CARTESIAN_POINT('Ctrl Pts',(16.0595421921667,-8.47078185490896,14.1481291139616));
#15580=CARTESIAN_POINT('Ctrl Pts',(16.2738279064524,-5.24156370981795,13.4110811449623));
#15581=CARTESIAN_POINT('Ctrl Pts',(16.4881136207381,-2.65193182212376,11.3459186275248));
#15582=CARTESIAN_POINT('Ctrl Pts',(16.7023993350239,-0.0622999344295592,
9.28075611008741));
#15583=CARTESIAN_POINT('Ctrl Pts',(16.9166850493096,1.37483734075912,6.2965098083465));
#15584=CARTESIAN_POINT('Ctrl Pts',(17.1309707635953,2.81197461594777,3.31226350660556));
#15585=CARTESIAN_POINT('Ctrl Pts',(17.345256477881,2.81197461594778,-2.10659534805265E-14));
#15586=CARTESIAN_POINT('Ctrl Pts',(17.5595421921667,2.81197461594776,-3.31226350660559));
#15587=CARTESIAN_POINT('Ctrl Pts',(17.7738279064524,1.37483734075912,-6.2965098083465));
#15588=CARTESIAN_POINT('Ctrl Pts',(17.9881136207381,-0.0622999344295592,
-9.28075611008743));
#15589=CARTESIAN_POINT('Ctrl Pts',(18.2023993350238,-2.65193182212374,-11.3459186275249));
#15590=CARTESIAN_POINT('Ctrl Pts',(18.4166850493096,-5.24156370981794,-13.4110811449623));
#15591=CARTESIAN_POINT('Ctrl Pts',(18.6309707635953,-8.47078185490896,-14.1481291139616));
#15592=CARTESIAN_POINT('Ctrl Pts',(18.845256477881,-11.7,-14.8851770829609));
#15593=CARTESIAN_POINT('Ctrl Pts',(19.0595421921667,-14.929218145091,-14.1481291139616));
#15594=CARTESIAN_POINT('Ctrl Pts',(19.2738279064524,-18.158436290182,-13.4110811449623));
#15595=CARTESIAN_POINT('Ctrl Pts',(19.4881136207381,-20.7480681778762,-11.3459186275249));
#15596=CARTESIAN_POINT('Ctrl Pts',(19.7023993350239,-23.3377000655704,-9.28075611008744));
#15597=CARTESIAN_POINT('Ctrl Pts',(19.9166850493096,-24.7748373407591,-6.29650980834651));
#15598=CARTESIAN_POINT('Ctrl Pts',(20.1309707635953,-26.2119746159478,-3.3122635066056));
#15599=CARTESIAN_POINT('Ctrl Pts',(20.345256477881,-26.2119746159477,-1.05329767402633E-14));
#15600=CARTESIAN_POINT('Ctrl Pts',(20.5595421921667,-26.2119746159478,3.31226350660556));
#15601=CARTESIAN_POINT('Ctrl Pts',(20.7738279064524,-24.7748373407591,6.29650980834649));
#15602=CARTESIAN_POINT('Ctrl Pts',(20.9881136207381,-23.3377000655704,9.28075611008741));
#15603=CARTESIAN_POINT('Ctrl Pts',(21.2023993350239,-20.7480681778762,11.3459186275248));
#15604=CARTESIAN_POINT('Ctrl Pts',(21.4166850493096,-18.158436290182,13.4110811449623));
#15605=CARTESIAN_POINT('Ctrl Pts',(21.6309707635953,-14.929218145091,14.1481291139616));
#15606=CARTESIAN_POINT('Ctrl Pts',(21.845256477881,-11.7,14.8851770829608));
#15607=CARTESIAN_POINT('Ctrl Pts',(22.0595421921667,-8.47078185490896,14.1481291139616));
#15608=CARTESIAN_POINT('Ctrl Pts',(22.2738279064524,-5.24156370981795,13.4110811449623));
#15609=CARTESIAN_POINT('Ctrl Pts',(22.4881136207381,-2.65193182212374,11.3459186275248));
#15610=CARTESIAN_POINT('Ctrl Pts',(22.7023993350238,-0.0622999344295592,
9.28075611008741));
#15611=CARTESIAN_POINT('Ctrl Pts',(22.9166850493096,1.37483734075912,6.2965098083465));
#15612=CARTESIAN_POINT('Ctrl Pts',(23.1309707635953,2.81197461594777,3.31226350660557));
#15613=CARTESIAN_POINT('Ctrl Pts',(23.345256477881,2.81197461594778,-7.02198449350884E-15));
#15614=CARTESIAN_POINT('Ctrl Pts',(-0.97049399036428,1.5411253090549,-6.93889390390723E-15));
#15615=CARTESIAN_POINT('Ctrl Pts',(-0.756208276078568,1.5411253090549,-3.02220044537404));
#15616=CARTESIAN_POINT('Ctrl Pts',(-0.541922561792853,0.229841679453259,
-5.74510895921687));
#15617=CARTESIAN_POINT('Ctrl Pts',(-0.327636847507138,-1.08144195014838,
-8.4680174730597));
#15618=CARTESIAN_POINT('Ctrl Pts',(-0.113351133221425,-3.4442934046707,
-10.3523286299233));
#15619=CARTESIAN_POINT('Ctrl Pts',(0.10093458106429,-5.80714485919302,-12.236639786787));
#15620=CARTESIAN_POINT('Ctrl Pts',(0.315220295350005,-8.75357242959651,
-12.9091426524948));
#15621=CARTESIAN_POINT('Ctrl Pts',(0.529506009635718,-11.7,-13.5816455182026));
#15622=CARTESIAN_POINT('Ctrl Pts',(0.743791723921435,-14.6464275704035,
-12.9091426524948));
#15623=CARTESIAN_POINT('Ctrl Pts',(0.958077438207147,-17.592855140807,-12.236639786787));
#15624=CARTESIAN_POINT('Ctrl Pts',(1.17236315249286,-19.9557065953293,-10.3523286299233));
#15625=CARTESIAN_POINT('Ctrl Pts',(1.38664886677857,-22.3185580498516,-8.4680174730597));
#15626=CARTESIAN_POINT('Ctrl Pts',(1.60093458106429,-23.6298416794532,-5.74510895921687));
#15627=CARTESIAN_POINT('Ctrl Pts',(1.81522029535,-24.9411253090549,-3.02220044537404));
#15628=CARTESIAN_POINT('Ctrl Pts',(2.02950600963572,-24.9411253090549,6.93889390390723E-15));
#15629=CARTESIAN_POINT('Ctrl Pts',(2.24379172392143,-24.9411253090549,3.02220044537403));
#15630=CARTESIAN_POINT('Ctrl Pts',(2.45807743820715,-23.6298416794532,5.74510895921686));
#15631=CARTESIAN_POINT('Ctrl Pts',(2.67236315249286,-22.3185580498516,8.4680174730597));
#15632=CARTESIAN_POINT('Ctrl Pts',(2.88664886677858,-19.9557065953293,10.3523286299233));
#15633=CARTESIAN_POINT('Ctrl Pts',(3.10093458106429,-17.592855140807,12.236639786787));
#15634=CARTESIAN_POINT('Ctrl Pts',(3.31522029535001,-14.6464275704035,12.9091426524948));
#15635=CARTESIAN_POINT('Ctrl Pts',(3.52950600963572,-11.7,13.5816455182026));
#15636=CARTESIAN_POINT('Ctrl Pts',(3.74379172392143,-8.7535724295965,12.9091426524948));
#15637=CARTESIAN_POINT('Ctrl Pts',(3.95807743820715,-5.80714485919301,12.236639786787));
#15638=CARTESIAN_POINT('Ctrl Pts',(4.17236315249286,-3.4442934046707,10.3523286299233));
#15639=CARTESIAN_POINT('Ctrl Pts',(4.38664886677858,-1.08144195014837,8.46801747305969));
#15640=CARTESIAN_POINT('Ctrl Pts',(4.60093458106429,0.229841679453252,5.74510895921686));
#15641=CARTESIAN_POINT('Ctrl Pts',(4.81522029535,1.5411253090549,3.02220044537404));
#15642=CARTESIAN_POINT('Ctrl Pts',(5.02950600963572,1.5411253090549,0.));
#15643=CARTESIAN_POINT('Ctrl Pts',(5.24379172392143,1.5411253090549,-3.02220044537404));
#15644=CARTESIAN_POINT('Ctrl Pts',(5.45807743820715,0.229841679453252,-5.74510895921687));
#15645=CARTESIAN_POINT('Ctrl Pts',(5.67236315249286,-1.08144195014837,-8.4680174730597));
#15646=CARTESIAN_POINT('Ctrl Pts',(5.88664886677858,-3.4442934046707,-10.3523286299233));
#15647=CARTESIAN_POINT('Ctrl Pts',(6.10093458106429,-5.80714485919301,-12.236639786787));
#15648=CARTESIAN_POINT('Ctrl Pts',(6.31522029535001,-8.75357242959651,-12.9091426524948));
#15649=CARTESIAN_POINT('Ctrl Pts',(6.52950600963572,-11.7,-13.5816455182026));
#15650=CARTESIAN_POINT('Ctrl Pts',(6.74379172392144,-14.6464275704035,-12.9091426524948));
#15651=CARTESIAN_POINT('Ctrl Pts',(6.95807743820715,-17.592855140807,-12.236639786787));
#15652=CARTESIAN_POINT('Ctrl Pts',(7.17236315249286,-19.9557065953293,-10.3523286299233));
#15653=CARTESIAN_POINT('Ctrl Pts',(7.38664886677858,-22.3185580498516,-8.4680174730597));
#15654=CARTESIAN_POINT('Ctrl Pts',(7.60093458106429,-23.6298416794532,-5.74510895921687));
#15655=CARTESIAN_POINT('Ctrl Pts',(7.81522029535,-24.9411253090549,-3.02220044537404));
#15656=CARTESIAN_POINT('Ctrl Pts',(8.02950600963572,-24.9411253090549,-6.93889390390723E-15));
#15657=CARTESIAN_POINT('Ctrl Pts',(8.24379172392143,-24.9411253090549,3.02220044537402));
#15658=CARTESIAN_POINT('Ctrl Pts',(8.45807743820715,-23.6298416794532,5.74510895921685));
#15659=CARTESIAN_POINT('Ctrl Pts',(8.67236315249286,-22.3185580498516,8.4680174730597));
#15660=CARTESIAN_POINT('Ctrl Pts',(8.88664886677858,-19.9557065953293,10.3523286299233));
#15661=CARTESIAN_POINT('Ctrl Pts',(9.10093458106429,-17.592855140807,12.236639786787));
#15662=CARTESIAN_POINT('Ctrl Pts',(9.31522029535001,-14.6464275704035,12.9091426524948));
#15663=CARTESIAN_POINT('Ctrl Pts',(9.52950600963572,-11.7,13.5816455182026));
#15664=CARTESIAN_POINT('Ctrl Pts',(9.74379172392144,-8.75357242959651,12.9091426524948));
#15665=CARTESIAN_POINT('Ctrl Pts',(9.95807743820714,-5.80714485919302,12.236639786787));
#15666=CARTESIAN_POINT('Ctrl Pts',(10.1723631524929,-3.4442934046707,10.3523286299233));
#15667=CARTESIAN_POINT('Ctrl Pts',(10.3866488667786,-1.08144195014837,8.4680174730597));
#15668=CARTESIAN_POINT('Ctrl Pts',(10.6009345810643,0.229841679453252,5.74510895921686));
#15669=CARTESIAN_POINT('Ctrl Pts',(10.81522029535,1.5411253090549,3.02220044537402));
#15670=CARTESIAN_POINT('Ctrl Pts',(11.0295060096357,1.5411253090549,6.93889390390723E-15));
#15671=CARTESIAN_POINT('Ctrl Pts',(11.2437917239214,1.54112530905489,-3.02220044537404));
#15672=CARTESIAN_POINT('Ctrl Pts',(11.4580774382071,0.229841679453259,-5.74510895921686));
#15673=CARTESIAN_POINT('Ctrl Pts',(11.6723631524929,-1.08144195014837,-8.4680174730597));
#15674=CARTESIAN_POINT('Ctrl Pts',(11.8866488667786,-3.4442934046707,-10.3523286299233));
#15675=CARTESIAN_POINT('Ctrl Pts',(12.1009345810643,-5.80714485919302,-12.236639786787));
#15676=CARTESIAN_POINT('Ctrl Pts',(12.31522029535,-8.75357242959649,-12.9091426524948));
#15677=CARTESIAN_POINT('Ctrl Pts',(12.5295060096357,-11.7,-13.5816455182026));
#15678=CARTESIAN_POINT('Ctrl Pts',(12.7437917239214,-14.6464275704035,-12.9091426524948));
#15679=CARTESIAN_POINT('Ctrl Pts',(12.9580774382071,-17.592855140807,-12.236639786787));
#15680=CARTESIAN_POINT('Ctrl Pts',(13.1723631524929,-19.9557065953293,-10.3523286299233));
#15681=CARTESIAN_POINT('Ctrl Pts',(13.3866488667786,-22.3185580498516,-8.4680174730597));
#15682=CARTESIAN_POINT('Ctrl Pts',(13.6009345810643,-23.6298416794532,-5.74510895921687));
#15683=CARTESIAN_POINT('Ctrl Pts',(13.81522029535,-24.9411253090549,-3.02220044537403));
#15684=CARTESIAN_POINT('Ctrl Pts',(14.0295060096357,-24.9411253090549,-6.93889390390723E-15));
#15685=CARTESIAN_POINT('Ctrl Pts',(14.2437917239214,-24.9411253090549,3.02220044537403));
#15686=CARTESIAN_POINT('Ctrl Pts',(14.4580774382072,-23.6298416794532,5.74510895921685));
#15687=CARTESIAN_POINT('Ctrl Pts',(14.6723631524929,-22.3185580498516,8.46801747305969));
#15688=CARTESIAN_POINT('Ctrl Pts',(14.8866488667786,-19.9557065953293,10.3523286299233));
#15689=CARTESIAN_POINT('Ctrl Pts',(15.1009345810643,-17.592855140807,12.236639786787));
#15690=CARTESIAN_POINT('Ctrl Pts',(15.31522029535,-14.6464275704035,12.9091426524948));
#15691=CARTESIAN_POINT('Ctrl Pts',(15.5295060096357,-11.7,13.5816455182026));
#15692=CARTESIAN_POINT('Ctrl Pts',(15.7437917239214,-8.75357242959651,12.9091426524948));
#15693=CARTESIAN_POINT('Ctrl Pts',(15.9580774382071,-5.80714485919302,12.236639786787));
#15694=CARTESIAN_POINT('Ctrl Pts',(16.1723631524929,-3.4442934046707,10.3523286299233));
#15695=CARTESIAN_POINT('Ctrl Pts',(16.3866488667786,-1.08144195014837,8.46801747305969));
#15696=CARTESIAN_POINT('Ctrl Pts',(16.6009345810643,0.229841679453266,5.74510895921686));
#15697=CARTESIAN_POINT('Ctrl Pts',(16.81522029535,1.5411253090549,3.02220044537404));
#15698=CARTESIAN_POINT('Ctrl Pts',(17.0295060096357,1.5411253090549,-2.08166817117217E-14));
#15699=CARTESIAN_POINT('Ctrl Pts',(17.2437917239214,1.5411253090549,-3.02220044537405));
#15700=CARTESIAN_POINT('Ctrl Pts',(17.4580774382072,0.229841679453266,-5.74510895921688));
#15701=CARTESIAN_POINT('Ctrl Pts',(17.6723631524929,-1.08144195014837,-8.46801747305971));
#15702=CARTESIAN_POINT('Ctrl Pts',(17.8866488667786,-3.44429340467071,-10.3523286299233));
#15703=CARTESIAN_POINT('Ctrl Pts',(18.1009345810643,-5.80714485919302,-12.236639786787));
#15704=CARTESIAN_POINT('Ctrl Pts',(18.31522029535,-8.75357242959651,-12.9091426524948));
#15705=CARTESIAN_POINT('Ctrl Pts',(18.5295060096357,-11.7,-13.5816455182026));
#15706=CARTESIAN_POINT('Ctrl Pts',(18.7437917239214,-14.6464275704035,-12.9091426524948));
#15707=CARTESIAN_POINT('Ctrl Pts',(18.9580774382071,-17.592855140807,-12.236639786787));
#15708=CARTESIAN_POINT('Ctrl Pts',(19.1723631524929,-19.9557065953293,-10.3523286299233));
#15709=CARTESIAN_POINT('Ctrl Pts',(19.3866488667786,-22.3185580498516,-8.4680174730597));
#15710=CARTESIAN_POINT('Ctrl Pts',(19.6009345810643,-23.6298416794532,-5.74510895921687));
#15711=CARTESIAN_POINT('Ctrl Pts',(19.81522029535,-24.9411253090549,-3.02220044537404));
#15712=CARTESIAN_POINT('Ctrl Pts',(20.0295060096357,-24.9411253090549,0.));
#15713=CARTESIAN_POINT('Ctrl Pts',(20.2437917239214,-24.9411253090549,3.02220044537403));
#15714=CARTESIAN_POINT('Ctrl Pts',(20.4580774382071,-23.6298416794532,5.74510895921685));
#15715=CARTESIAN_POINT('Ctrl Pts',(20.6723631524929,-22.3185580498516,8.46801747305969));
#15716=CARTESIAN_POINT('Ctrl Pts',(20.8866488667786,-19.9557065953293,10.3523286299233));
#15717=CARTESIAN_POINT('Ctrl Pts',(21.1009345810643,-17.5928551408069,12.236639786787));
#15718=CARTESIAN_POINT('Ctrl Pts',(21.31522029535,-14.6464275704035,12.9091426524948));
#15719=CARTESIAN_POINT('Ctrl Pts',(21.5295060096357,-11.7,13.5816455182026));
#15720=CARTESIAN_POINT('Ctrl Pts',(21.7437917239214,-8.75357242959651,12.9091426524948));
#15721=CARTESIAN_POINT('Ctrl Pts',(21.9580774382071,-5.80714485919301,12.236639786787));
#15722=CARTESIAN_POINT('Ctrl Pts',(22.1723631524929,-3.4442934046707,10.3523286299233));
#15723=CARTESIAN_POINT('Ctrl Pts',(22.3866488667786,-1.08144195014837,8.4680174730597));
#15724=CARTESIAN_POINT('Ctrl Pts',(22.6009345810643,0.229841679453259,5.74510895921686));
#15725=CARTESIAN_POINT('Ctrl Pts',(22.81522029535,1.54112530905491,3.02220044537404));
#15726=CARTESIAN_POINT('Ctrl Pts',(23.0295060096357,1.5411253090549,0.));
#15727=CARTESIAN_POINT('',(0.970493990364278,1.5411253090549,-1.38777878078145E-14));
#15728=CARTESIAN_POINT('Origin',(-2.60208521396521E-15,1.30000000000001,
-2.08166817117217E-14));
#15729=CARTESIAN_POINT('Ctrl Pts',(0.970493990364278,1.5411253090549,-1.38777878078145E-14));
#15730=CARTESIAN_POINT('Ctrl Pts',(1.18477970464999,1.54112530905491,-3.02220044537403));
#15731=CARTESIAN_POINT('Ctrl Pts',(1.39906541893571,0.229841679453259,-5.74510895921686));
#15732=CARTESIAN_POINT('Ctrl Pts',(1.61335113322142,-1.08144195014838,-8.4680174730597));
#15733=CARTESIAN_POINT('Ctrl Pts',(1.82763684750713,-3.44429340467071,-10.3523286299233));
#15734=CARTESIAN_POINT('Ctrl Pts',(2.04192256179285,-5.80714485919301,-12.236639786787));
#15735=CARTESIAN_POINT('Ctrl Pts',(2.25620827607856,-8.75357242959651,-12.9091426524948));
#15736=CARTESIAN_POINT('Ctrl Pts',(2.47049399036428,-11.7,-13.5816455182026));
#15737=CARTESIAN_POINT('Ctrl Pts',(2.68477970464999,-14.6464275704035,-12.9091426524948));
#15738=CARTESIAN_POINT('Ctrl Pts',(2.89906541893571,-17.592855140807,-12.236639786787));
#15739=CARTESIAN_POINT('Ctrl Pts',(3.11335113322142,-19.9557065953293,-10.3523286299233));
#15740=CARTESIAN_POINT('Ctrl Pts',(3.32763684750713,-22.3185580498516,-8.4680174730597));
#15741=CARTESIAN_POINT('Ctrl Pts',(3.54192256179285,-23.6298416794532,-5.74510895921686));
#15742=CARTESIAN_POINT('Ctrl Pts',(3.75620827607856,-24.9411253090549,-3.02220044537403));
#15743=CARTESIAN_POINT('Ctrl Pts',(3.97049399036428,-24.9411253090549,3.46944695195361E-15));
#15744=CARTESIAN_POINT('Ctrl Pts',(4.18477970464999,-24.9411253090549,3.02220044537403));
#15745=CARTESIAN_POINT('Ctrl Pts',(4.39906541893571,-23.6298416794532,5.74510895921686));
#15746=CARTESIAN_POINT('Ctrl Pts',(4.61335113322142,-22.3185580498516,8.46801747305969));
#15747=CARTESIAN_POINT('Ctrl Pts',(4.82763684750714,-19.9557065953293,10.3523286299233));
#15748=CARTESIAN_POINT('Ctrl Pts',(5.04192256179285,-17.592855140807,12.2366397867869));
#15749=CARTESIAN_POINT('Ctrl Pts',(5.25620827607856,-14.6464275704035,12.9091426524948));
#15750=CARTESIAN_POINT('Ctrl Pts',(5.47049399036428,-11.7,13.5816455182026));
#15751=CARTESIAN_POINT('Ctrl Pts',(5.68477970464999,-8.75357242959651,12.9091426524948));
#15752=CARTESIAN_POINT('Ctrl Pts',(5.89906541893571,-5.80714485919302,12.236639786787));
#15753=CARTESIAN_POINT('Ctrl Pts',(6.11335113322142,-3.4442934046707,10.3523286299233));
#15754=CARTESIAN_POINT('Ctrl Pts',(6.32763684750713,-1.08144195014838,8.4680174730597));
#15755=CARTESIAN_POINT('Ctrl Pts',(6.54192256179285,0.229841679453252,5.74510895921686));
#15756=CARTESIAN_POINT('Ctrl Pts',(6.75620827607856,1.5411253090549,3.02220044537404));
#15757=CARTESIAN_POINT('Ctrl Pts',(6.97049399036428,1.5411253090549,-1.38777878078145E-14));
#15758=CARTESIAN_POINT('Ctrl Pts',(7.18477970464999,1.5411253090549,-3.02220044537404));
#15759=CARTESIAN_POINT('Ctrl Pts',(7.39906541893571,0.229841679453259,-5.74510895921689));
#15760=CARTESIAN_POINT('Ctrl Pts',(7.61335113322142,-1.08144195014838,-8.46801747305971));
#15761=CARTESIAN_POINT('Ctrl Pts',(7.82763684750713,-3.4442934046707,-10.3523286299233));
#15762=CARTESIAN_POINT('Ctrl Pts',(8.04192256179285,-5.80714485919302,-12.236639786787));
#15763=CARTESIAN_POINT('Ctrl Pts',(8.25620827607856,-8.75357242959651,-12.9091426524948));
#15764=CARTESIAN_POINT('Ctrl Pts',(8.47049399036428,-11.7,-13.5816455182026));
#15765=CARTESIAN_POINT('Ctrl Pts',(8.68477970464999,-14.6464275704035,-12.9091426524948));
#15766=CARTESIAN_POINT('Ctrl Pts',(8.89906541893571,-17.592855140807,-12.236639786787));
#15767=CARTESIAN_POINT('Ctrl Pts',(9.11335113322142,-19.9557065953293,-10.3523286299233));
#15768=CARTESIAN_POINT('Ctrl Pts',(9.32763684750714,-22.3185580498516,-8.4680174730597));
#15769=CARTESIAN_POINT('Ctrl Pts',(9.54192256179285,-23.6298416794532,-5.74510895921687));
#15770=CARTESIAN_POINT('Ctrl Pts',(9.75620827607856,-24.9411253090549,-3.02220044537404));
#15771=CARTESIAN_POINT('Ctrl Pts',(9.97049399036428,-24.9411253090549,-6.93889390390723E-15));
#15772=CARTESIAN_POINT('Ctrl Pts',(10.18477970465,-24.9411253090549,3.02220044537403));
#15773=CARTESIAN_POINT('Ctrl Pts',(10.3990654189357,-23.6298416794532,5.74510895921686));
#15774=CARTESIAN_POINT('Ctrl Pts',(10.6133511332214,-22.3185580498516,8.4680174730597));
#15775=CARTESIAN_POINT('Ctrl Pts',(10.8276368475071,-19.9557065953293,10.3523286299233));
#15776=CARTESIAN_POINT('Ctrl Pts',(11.0419225617928,-17.592855140807,12.236639786787));
#15777=CARTESIAN_POINT('Ctrl Pts',(11.2562082760786,-14.6464275704035,12.9091426524948));
#15778=CARTESIAN_POINT('Ctrl Pts',(11.4704939903643,-11.7,13.5816455182026));
#15779=CARTESIAN_POINT('Ctrl Pts',(11.68477970465,-8.75357242959651,12.9091426524948));
#15780=CARTESIAN_POINT('Ctrl Pts',(11.8990654189357,-5.80714485919301,12.236639786787));
#15781=CARTESIAN_POINT('Ctrl Pts',(12.1133511332214,-3.4442934046707,10.3523286299233));
#15782=CARTESIAN_POINT('Ctrl Pts',(12.3276368475071,-1.08144195014836,8.4680174730597));
#15783=CARTESIAN_POINT('Ctrl Pts',(12.5419225617929,0.229841679453266,5.74510895921686));
#15784=CARTESIAN_POINT('Ctrl Pts',(12.7562082760786,1.5411253090549,3.02220044537403));
#15785=CARTESIAN_POINT('Ctrl Pts',(12.9704939903643,1.5411253090549,-2.08166817117217E-14));
#15786=CARTESIAN_POINT('Ctrl Pts',(13.18477970465,1.5411253090549,-3.02220044537405));
#15787=CARTESIAN_POINT('Ctrl Pts',(13.3990654189357,0.229841679453252,-5.74510895921687));
#15788=CARTESIAN_POINT('Ctrl Pts',(13.6133511332214,-1.08144195014838,-8.46801747305971));
#15789=CARTESIAN_POINT('Ctrl Pts',(13.8276368475071,-3.44429340467069,-10.3523286299233));
#15790=CARTESIAN_POINT('Ctrl Pts',(14.0419225617929,-5.80714485919301,-12.236639786787));
#15791=CARTESIAN_POINT('Ctrl Pts',(14.2562082760786,-8.75357242959651,-12.9091426524948));
#15792=CARTESIAN_POINT('Ctrl Pts',(14.4704939903643,-11.7,-13.5816455182026));
#15793=CARTESIAN_POINT('Ctrl Pts',(14.68477970465,-14.6464275704035,-12.9091426524948));
#15794=CARTESIAN_POINT('Ctrl Pts',(14.8990654189357,-17.592855140807,-12.236639786787));
#15795=CARTESIAN_POINT('Ctrl Pts',(15.1133511332214,-19.9557065953293,-10.3523286299233));
#15796=CARTESIAN_POINT('Ctrl Pts',(15.3276368475071,-22.3185580498516,-8.46801747305969));
#15797=CARTESIAN_POINT('Ctrl Pts',(15.5419225617929,-23.6298416794532,-5.74510895921687));
#15798=CARTESIAN_POINT('Ctrl Pts',(15.7562082760786,-24.9411253090549,-3.02220044537403));
#15799=CARTESIAN_POINT('Ctrl Pts',(15.9704939903643,-24.9411253090549,-6.93889390390723E-15));
#15800=CARTESIAN_POINT('Ctrl Pts',(16.18477970465,-24.9411253090549,3.02220044537403));
#15801=CARTESIAN_POINT('Ctrl Pts',(16.3990654189357,-23.6298416794532,5.74510895921686));
#15802=CARTESIAN_POINT('Ctrl Pts',(16.6133511332214,-22.3185580498516,8.46801747305969));
#15803=CARTESIAN_POINT('Ctrl Pts',(16.8276368475071,-19.9557065953293,10.3523286299233));
#15804=CARTESIAN_POINT('Ctrl Pts',(17.0419225617928,-17.592855140807,12.236639786787));
#15805=CARTESIAN_POINT('Ctrl Pts',(17.2562082760786,-14.6464275704035,12.9091426524948));
#15806=CARTESIAN_POINT('Ctrl Pts',(17.4704939903643,-11.7,13.5816455182026));
#15807=CARTESIAN_POINT('Ctrl Pts',(17.68477970465,-8.75357242959651,12.9091426524948));
#15808=CARTESIAN_POINT('Ctrl Pts',(17.8990654189357,-5.80714485919301,12.236639786787));
#15809=CARTESIAN_POINT('Ctrl Pts',(18.1133511332214,-3.4442934046707,10.3523286299233));
#15810=CARTESIAN_POINT('Ctrl Pts',(18.3276368475071,-1.08144195014837,8.46801747305969));
#15811=CARTESIAN_POINT('Ctrl Pts',(18.5419225617928,0.229841679453252,5.74510895921686));
#15812=CARTESIAN_POINT('Ctrl Pts',(18.7562082760786,1.5411253090549,3.02220044537405));
#15813=CARTESIAN_POINT('Ctrl Pts',(18.9704939903643,1.5411253090549,-1.38777878078145E-14));
#15814=CARTESIAN_POINT('Ctrl Pts',(19.18477970465,1.5411253090549,-3.02220044537404));
#15815=CARTESIAN_POINT('Ctrl Pts',(19.3990654189357,0.229841679453259,-5.74510895921686));
#15816=CARTESIAN_POINT('Ctrl Pts',(19.6133511332214,-1.08144195014838,-8.4680174730597));
#15817=CARTESIAN_POINT('Ctrl Pts',(19.8276368475071,-3.4442934046707,-10.3523286299233));
#15818=CARTESIAN_POINT('Ctrl Pts',(20.0419225617929,-5.80714485919302,-12.236639786787));
#15819=CARTESIAN_POINT('Ctrl Pts',(20.2562082760786,-8.75357242959651,-12.9091426524948));
#15820=CARTESIAN_POINT('Ctrl Pts',(20.4704939903643,-11.7,-13.5816455182026));
#15821=CARTESIAN_POINT('Ctrl Pts',(20.68477970465,-14.6464275704035,-12.9091426524948));
#15822=CARTESIAN_POINT('Ctrl Pts',(20.8990654189357,-17.592855140807,-12.236639786787));
#15823=CARTESIAN_POINT('Ctrl Pts',(21.1133511332214,-19.9557065953293,-10.3523286299233));
#15824=CARTESIAN_POINT('Ctrl Pts',(21.3276368475071,-22.3185580498516,-8.4680174730597));
#15825=CARTESIAN_POINT('Ctrl Pts',(21.5419225617929,-23.6298416794532,-5.74510895921687));
#15826=CARTESIAN_POINT('Ctrl Pts',(21.7562082760786,-24.9411253090549,-3.02220044537404));
#15827=CARTESIAN_POINT('Ctrl Pts',(21.9704939903643,-24.9411253090549,-3.46944695195361E-15));
#15828=CARTESIAN_POINT('Ctrl Pts',(22.18477970465,-24.9411253090549,3.02220044537403));
#15829=CARTESIAN_POINT('Ctrl Pts',(22.3990654189357,-23.6298416794532,5.74510895921686));
#15830=CARTESIAN_POINT('Ctrl Pts',(22.6133511332214,-22.3185580498516,8.46801747305969));
#15831=CARTESIAN_POINT('Ctrl Pts',(22.8276368475071,-19.9557065953293,10.3523286299233));
#15832=CARTESIAN_POINT('Ctrl Pts',(23.0419225617928,-17.592855140807,12.236639786787));
#15833=CARTESIAN_POINT('Ctrl Pts',(23.2562082760786,-14.6464275704035,12.9091426524948));
#15834=CARTESIAN_POINT('Ctrl Pts',(23.4704939903643,-11.7,13.5816455182026));
#15835=CARTESIAN_POINT('Ctrl Pts',(23.68477970465,-8.75357242959651,12.9091426524948));
#15836=CARTESIAN_POINT('Ctrl Pts',(23.8990654189357,-5.80714485919302,12.236639786787));
#15837=CARTESIAN_POINT('Ctrl Pts',(24.1133511332214,-3.4442934046707,10.3523286299233));
#15838=CARTESIAN_POINT('Ctrl Pts',(24.3276368475071,-1.08144195014837,8.46801747305969));
#15839=CARTESIAN_POINT('Ctrl Pts',(24.5419225617928,0.229841679453252,5.74510895921686));
#15840=CARTESIAN_POINT('Ctrl Pts',(24.7562082760786,1.5411253090549,3.02220044537404));
#15841=CARTESIAN_POINT('Ctrl Pts',(24.9704939903643,1.5411253090549,0.));
#15842=CARTESIAN_POINT('Ctrl Pts',(1.9,-2.19999999999999,0.));
#15843=CARTESIAN_POINT('Ctrl Pts',(2.11428571428571,-2.19999999999999,-2.16831300670642));
#15844=CARTESIAN_POINT('Ctrl Pts',(2.32857142857143,-3.14079575492701,-4.12189552161681));
#15845=CARTESIAN_POINT('Ctrl Pts',(2.54285714285714,-4.08159150985404,-6.07547803652717));
#15846=CARTESIAN_POINT('Ctrl Pts',(2.75714285714286,-5.77684688234201,-7.42739908344628));
#15847=CARTESIAN_POINT('Ctrl Pts',(2.97142857142857,-7.47210225483002,-8.77932013036538));
#15848=CARTESIAN_POINT('Ctrl Pts',(3.18571428571428,-9.58605112741501,-9.26181516572732));
#15849=CARTESIAN_POINT('Ctrl Pts',(3.4,-11.7,-9.74431020108927));
#15850=CARTESIAN_POINT('Ctrl Pts',(3.61428571428571,-13.813948872585,-9.26181516572732));
#15851=CARTESIAN_POINT('Ctrl Pts',(3.82857142857143,-15.92789774517,-8.77932013036538));
#15852=CARTESIAN_POINT('Ctrl Pts',(4.04285714285714,-17.623153117658,-7.42739908344629));
#15853=CARTESIAN_POINT('Ctrl Pts',(4.25714285714286,-19.3184084901459,-6.07547803652718));
#15854=CARTESIAN_POINT('Ctrl Pts',(4.47142857142857,-20.259204245073,-4.12189552161681));
#15855=CARTESIAN_POINT('Ctrl Pts',(4.68571428571428,-21.2,-2.16831300670643));
#15856=CARTESIAN_POINT('Ctrl Pts',(4.9,-21.2,-6.93889390390723E-15));
#15857=CARTESIAN_POINT('Ctrl Pts',(5.11428571428571,-21.2,2.16831300670641));
#15858=CARTESIAN_POINT('Ctrl Pts',(5.32857142857143,-20.259204245073,4.12189552161679));
#15859=CARTESIAN_POINT('Ctrl Pts',(5.54285714285714,-19.3184084901459,6.07547803652717));
#15860=CARTESIAN_POINT('Ctrl Pts',(5.75714285714286,-17.623153117658,7.42739908344627));
#15861=CARTESIAN_POINT('Ctrl Pts',(5.97142857142857,-15.92789774517,8.77932013036537));
#15862=CARTESIAN_POINT('Ctrl Pts',(6.18571428571429,-13.813948872585,9.26181516572732));
#15863=CARTESIAN_POINT('Ctrl Pts',(6.4,-11.7,9.74431020108925));
#15864=CARTESIAN_POINT('Ctrl Pts',(6.61428571428571,-9.586051127415,9.26181516572731));
#15865=CARTESIAN_POINT('Ctrl Pts',(6.82857142857143,-7.47210225483002,8.77932013036537));
#15866=CARTESIAN_POINT('Ctrl Pts',(7.04285714285714,-5.77684688234203,7.42739908344628));
#15867=CARTESIAN_POINT('Ctrl Pts',(7.25714285714285,-4.08159150985402,6.07547803652718));
#15868=CARTESIAN_POINT('Ctrl Pts',(7.47142857142857,-3.14079575492702,4.12189552161681));
#15869=CARTESIAN_POINT('Ctrl Pts',(7.68571428571429,-2.2,2.16831300670643));
#15870=CARTESIAN_POINT('Ctrl Pts',(7.9,-2.19999999999999,6.93889390390723E-15));
#15871=CARTESIAN_POINT('Ctrl Pts',(8.11428571428571,-2.19999999999999,-2.16831300670641));
#15872=CARTESIAN_POINT('Ctrl Pts',(8.32857142857143,-3.14079575492703,-4.1218955216168));
#15873=CARTESIAN_POINT('Ctrl Pts',(8.54285714285714,-4.08159150985404,-6.07547803652717));
#15874=CARTESIAN_POINT('Ctrl Pts',(8.75714285714286,-5.77684688234202,-7.42739908344627));
#15875=CARTESIAN_POINT('Ctrl Pts',(8.97142857142857,-7.47210225483002,-8.77932013036538));
#15876=CARTESIAN_POINT('Ctrl Pts',(9.18571428571429,-9.58605112741501,-9.26181516572732));
#15877=CARTESIAN_POINT('Ctrl Pts',(9.4,-11.7,-9.74431020108925));
#15878=CARTESIAN_POINT('Ctrl Pts',(9.61428571428572,-13.813948872585,-9.26181516572732));
#15879=CARTESIAN_POINT('Ctrl Pts',(9.82857142857143,-15.92789774517,-8.77932013036538));
#15880=CARTESIAN_POINT('Ctrl Pts',(10.0428571428571,-17.6231531176579,-7.42739908344629));
#15881=CARTESIAN_POINT('Ctrl Pts',(10.2571428571429,-19.3184084901459,-6.07547803652717));
#15882=CARTESIAN_POINT('Ctrl Pts',(10.4714285714286,-20.259204245073,-4.1218955216168));
#15883=CARTESIAN_POINT('Ctrl Pts',(10.6857142857143,-21.2,-2.16831300670643));
#15884=CARTESIAN_POINT('Ctrl Pts',(10.9,-21.2,-6.93889390390723E-15));
#15885=CARTESIAN_POINT('Ctrl Pts',(11.1142857142857,-21.2,2.16831300670642));
#15886=CARTESIAN_POINT('Ctrl Pts',(11.3285714285714,-20.259204245073,4.12189552161679));
#15887=CARTESIAN_POINT('Ctrl Pts',(11.5428571428571,-19.3184084901459,6.07547803652716));
#15888=CARTESIAN_POINT('Ctrl Pts',(11.7571428571429,-17.623153117658,7.42739908344626));
#15889=CARTESIAN_POINT('Ctrl Pts',(11.9714285714286,-15.92789774517,8.77932013036537));
#15890=CARTESIAN_POINT('Ctrl Pts',(12.1857142857143,-13.813948872585,9.26181516572731));
#15891=CARTESIAN_POINT('Ctrl Pts',(12.4,-11.7,9.74431020108925));
#15892=CARTESIAN_POINT('Ctrl Pts',(12.6142857142857,-9.58605112741501,9.26181516572731));
#15893=CARTESIAN_POINT('Ctrl Pts',(12.8285714285714,-7.47210225483002,8.77932013036537));
#15894=CARTESIAN_POINT('Ctrl Pts',(13.0428571428571,-5.77684688234202,7.42739908344626));
#15895=CARTESIAN_POINT('Ctrl Pts',(13.2571428571429,-4.08159150985402,6.07547803652717));
#15896=CARTESIAN_POINT('Ctrl Pts',(13.4714285714286,-3.14079575492703,4.1218955216168));
#15897=CARTESIAN_POINT('Ctrl Pts',(13.6857142857143,-2.2,2.16831300670642));
#15898=CARTESIAN_POINT('Ctrl Pts',(13.9,-2.2,-6.93889390390723E-15));
#15899=CARTESIAN_POINT('Ctrl Pts',(14.1142857142857,-2.19999999999999,-2.16831300670644));
#15900=CARTESIAN_POINT('Ctrl Pts',(14.3285714285714,-3.14079575492702,-4.1218955216168));
#15901=CARTESIAN_POINT('Ctrl Pts',(14.5428571428571,-4.08159150985404,-6.07547803652717));
#15902=CARTESIAN_POINT('Ctrl Pts',(14.7571428571429,-5.77684688234202,-7.42739908344627));
#15903=CARTESIAN_POINT('Ctrl Pts',(14.9714285714286,-7.47210225483002,-8.77932013036538));
#15904=CARTESIAN_POINT('Ctrl Pts',(15.1857142857143,-9.58605112741499,-9.26181516572731));
#15905=CARTESIAN_POINT('Ctrl Pts',(15.4,-11.7,-9.74431020108925));
#15906=CARTESIAN_POINT('Ctrl Pts',(15.6142857142857,-13.813948872585,-9.26181516572732));
#15907=CARTESIAN_POINT('Ctrl Pts',(15.8285714285714,-15.92789774517,-8.77932013036537));
#15908=CARTESIAN_POINT('Ctrl Pts',(16.0428571428571,-17.6231531176579,-7.42739908344629));
#15909=CARTESIAN_POINT('Ctrl Pts',(16.2571428571428,-19.3184084901459,-6.07547803652718));
#15910=CARTESIAN_POINT('Ctrl Pts',(16.4714285714286,-20.259204245073,-4.12189552161682));
#15911=CARTESIAN_POINT('Ctrl Pts',(16.6857142857143,-21.2,-2.16831300670643));
#15912=CARTESIAN_POINT('Ctrl Pts',(16.9,-21.2,0.));
#15913=CARTESIAN_POINT('Ctrl Pts',(17.1142857142857,-21.2,2.16831300670642));
#15914=CARTESIAN_POINT('Ctrl Pts',(17.3285714285714,-20.259204245073,4.12189552161679));
#15915=CARTESIAN_POINT('Ctrl Pts',(17.5428571428572,-19.318408490146,6.07547803652717));
#15916=CARTESIAN_POINT('Ctrl Pts',(17.7571428571429,-17.623153117658,7.42739908344627));
#15917=CARTESIAN_POINT('Ctrl Pts',(17.9714285714286,-15.92789774517,8.77932013036537));
#15918=CARTESIAN_POINT('Ctrl Pts',(18.1857142857143,-13.813948872585,9.26181516572731));
#15919=CARTESIAN_POINT('Ctrl Pts',(18.4,-11.7,9.74431020108925));
#15920=CARTESIAN_POINT('Ctrl Pts',(18.6142857142857,-9.58605112741501,9.26181516572731));
#15921=CARTESIAN_POINT('Ctrl Pts',(18.8285714285714,-7.47210225483001,8.77932013036538));
#15922=CARTESIAN_POINT('Ctrl Pts',(19.0428571428571,-5.77684688234202,7.42739908344627));
#15923=CARTESIAN_POINT('Ctrl Pts',(19.2571428571429,-4.08159150985404,6.07547803652718));
#15924=CARTESIAN_POINT('Ctrl Pts',(19.4714285714286,-3.14079575492701,4.12189552161679));
#15925=CARTESIAN_POINT('Ctrl Pts',(19.6857142857143,-2.20000000000001,2.16831300670641));
#15926=CARTESIAN_POINT('Ctrl Pts',(19.9,-2.2,-1.38777878078145E-14));
#15927=CARTESIAN_POINT('Ctrl Pts',(20.1142857142857,-2.2,-2.16831300670642));
#15928=CARTESIAN_POINT('Ctrl Pts',(20.3285714285714,-3.14079575492703,-4.12189552161681));
#15929=CARTESIAN_POINT('Ctrl Pts',(20.5428571428571,-4.08159150985403,-6.07547803652718));
#15930=CARTESIAN_POINT('Ctrl Pts',(20.7571428571428,-5.77684688234203,-7.42739908344629));
#15931=CARTESIAN_POINT('Ctrl Pts',(20.9714285714286,-7.47210225483002,-8.77932013036538));
#15932=CARTESIAN_POINT('Ctrl Pts',(21.1857142857143,-9.58605112741501,-9.26181516572732));
#15933=CARTESIAN_POINT('Ctrl Pts',(21.4,-11.7,-9.74431020108924));
#15934=CARTESIAN_POINT('Ctrl Pts',(21.6142857142857,-13.813948872585,-9.26181516572731));
#15935=CARTESIAN_POINT('Ctrl Pts',(21.8285714285714,-15.92789774517,-8.77932013036537));
#15936=CARTESIAN_POINT('Ctrl Pts',(22.0428571428571,-17.6231531176579,-7.42739908344628));
#15937=CARTESIAN_POINT('Ctrl Pts',(22.2571428571429,-19.3184084901459,-6.07547803652717));
#15938=CARTESIAN_POINT('Ctrl Pts',(22.4714285714286,-20.259204245073,-4.12189552161681));
#15939=CARTESIAN_POINT('Ctrl Pts',(22.6857142857143,-21.2,-2.16831300670643));
#15940=CARTESIAN_POINT('Ctrl Pts',(22.9,-21.2,-1.04083408558608E-14));
#15941=CARTESIAN_POINT('Ctrl Pts',(23.1142857142857,-21.2,2.16831300670641));
#15942=CARTESIAN_POINT('Ctrl Pts',(23.3285714285714,-20.259204245073,4.1218955216168));
#15943=CARTESIAN_POINT('Ctrl Pts',(23.5428571428571,-19.3184084901459,6.07547803652717));
#15944=CARTESIAN_POINT('Ctrl Pts',(23.7571428571429,-17.623153117658,7.42739908344627));
#15945=CARTESIAN_POINT('Ctrl Pts',(23.9714285714286,-15.92789774517,8.77932013036537));
#15946=CARTESIAN_POINT('Ctrl Pts',(24.1857142857143,-13.813948872585,9.26181516572731));
#15947=CARTESIAN_POINT('Ctrl Pts',(24.4,-11.7,9.74431020108925));
#15948=CARTESIAN_POINT('Ctrl Pts',(24.6142857142857,-9.58605112741501,9.26181516572731));
#15949=CARTESIAN_POINT('Ctrl Pts',(24.8285714285714,-7.47210225483001,8.77932013036537));
#15950=CARTESIAN_POINT('Ctrl Pts',(25.0428571428571,-5.77684688234203,7.42739908344628));
#15951=CARTESIAN_POINT('Ctrl Pts',(25.2571428571429,-4.08159150985402,6.07547803652716));
#15952=CARTESIAN_POINT('Ctrl Pts',(25.4714285714286,-3.14079575492702,4.1218955216168));
#15953=CARTESIAN_POINT('Ctrl Pts',(25.6857142857143,-2.2,2.16831300670643));
#15954=CARTESIAN_POINT('Ctrl Pts',(25.9,-2.20000000000001,-1.38777878078145E-14));
#15955=CARTESIAN_POINT('Ctrl Pts',(0.970493990364278,1.5411253090549,-1.38777878078145E-14));
#15956=CARTESIAN_POINT('Ctrl Pts',(1.18477970464999,1.54112530905491,-3.02220044537403));
#15957=CARTESIAN_POINT('Ctrl Pts',(1.39906541893571,0.229841679453259,-5.74510895921686));
#15958=CARTESIAN_POINT('Ctrl Pts',(1.61335113322142,-1.08144195014838,-8.4680174730597));
#15959=CARTESIAN_POINT('Ctrl Pts',(1.82763684750713,-3.44429340467071,-10.3523286299233));
#15960=CARTESIAN_POINT('Ctrl Pts',(2.04192256179285,-5.80714485919301,-12.236639786787));
#15961=CARTESIAN_POINT('Ctrl Pts',(2.25620827607856,-8.75357242959651,-12.9091426524948));
#15962=CARTESIAN_POINT('Ctrl Pts',(2.47049399036428,-11.7,-13.5816455182026));
#15963=CARTESIAN_POINT('Ctrl Pts',(2.68477970464999,-14.6464275704035,-12.9091426524948));
#15964=CARTESIAN_POINT('Ctrl Pts',(2.89906541893571,-17.592855140807,-12.236639786787));
#15965=CARTESIAN_POINT('Ctrl Pts',(3.11335113322142,-19.9557065953293,-10.3523286299233));
#15966=CARTESIAN_POINT('Ctrl Pts',(3.32763684750713,-22.3185580498516,-8.4680174730597));
#15967=CARTESIAN_POINT('Ctrl Pts',(3.54192256179285,-23.6298416794532,-5.74510895921686));
#15968=CARTESIAN_POINT('Ctrl Pts',(3.75620827607856,-24.9411253090549,-3.02220044537403));
#15969=CARTESIAN_POINT('Ctrl Pts',(3.97049399036428,-24.9411253090549,3.46944695195361E-15));
#15970=CARTESIAN_POINT('Ctrl Pts',(4.18477970464999,-24.9411253090549,3.02220044537403));
#15971=CARTESIAN_POINT('Ctrl Pts',(4.39906541893571,-23.6298416794532,5.74510895921686));
#15972=CARTESIAN_POINT('Ctrl Pts',(4.61335113322142,-22.3185580498516,8.46801747305969));
#15973=CARTESIAN_POINT('Ctrl Pts',(4.82763684750714,-19.9557065953293,10.3523286299233));
#15974=CARTESIAN_POINT('Ctrl Pts',(5.04192256179285,-17.592855140807,12.2366397867869));
#15975=CARTESIAN_POINT('Ctrl Pts',(5.25620827607856,-14.6464275704035,12.9091426524948));
#15976=CARTESIAN_POINT('Ctrl Pts',(5.47049399036428,-11.7,13.5816455182026));
#15977=CARTESIAN_POINT('Ctrl Pts',(5.68477970464999,-8.75357242959651,12.9091426524948));
#15978=CARTESIAN_POINT('Ctrl Pts',(5.89906541893571,-5.80714485919302,12.236639786787));
#15979=CARTESIAN_POINT('Ctrl Pts',(6.11335113322142,-3.4442934046707,10.3523286299233));
#15980=CARTESIAN_POINT('Ctrl Pts',(6.32763684750713,-1.08144195014838,8.4680174730597));
#15981=CARTESIAN_POINT('Ctrl Pts',(6.54192256179285,0.229841679453252,5.74510895921686));
#15982=CARTESIAN_POINT('Ctrl Pts',(6.75620827607856,1.5411253090549,3.02220044537404));
#15983=CARTESIAN_POINT('Ctrl Pts',(6.97049399036428,1.5411253090549,-1.38777878078145E-14));
#15984=CARTESIAN_POINT('Ctrl Pts',(7.18477970464999,1.5411253090549,-3.02220044537404));
#15985=CARTESIAN_POINT('Ctrl Pts',(7.39906541893571,0.229841679453259,-5.74510895921689));
#15986=CARTESIAN_POINT('Ctrl Pts',(7.61335113322142,-1.08144195014838,-8.46801747305971));
#15987=CARTESIAN_POINT('Ctrl Pts',(7.82763684750713,-3.4442934046707,-10.3523286299233));
#15988=CARTESIAN_POINT('Ctrl Pts',(8.04192256179285,-5.80714485919302,-12.236639786787));
#15989=CARTESIAN_POINT('Ctrl Pts',(8.25620827607856,-8.75357242959651,-12.9091426524948));
#15990=CARTESIAN_POINT('Ctrl Pts',(8.47049399036428,-11.7,-13.5816455182026));
#15991=CARTESIAN_POINT('Ctrl Pts',(8.68477970464999,-14.6464275704035,-12.9091426524948));
#15992=CARTESIAN_POINT('Ctrl Pts',(8.89906541893571,-17.592855140807,-12.236639786787));
#15993=CARTESIAN_POINT('Ctrl Pts',(9.11335113322142,-19.9557065953293,-10.3523286299233));
#15994=CARTESIAN_POINT('Ctrl Pts',(9.32763684750714,-22.3185580498516,-8.4680174730597));
#15995=CARTESIAN_POINT('Ctrl Pts',(9.54192256179285,-23.6298416794532,-5.74510895921687));
#15996=CARTESIAN_POINT('Ctrl Pts',(9.75620827607856,-24.9411253090549,-3.02220044537404));
#15997=CARTESIAN_POINT('Ctrl Pts',(9.97049399036428,-24.9411253090549,-6.93889390390723E-15));
#15998=CARTESIAN_POINT('Ctrl Pts',(10.18477970465,-24.9411253090549,3.02220044537403));
#15999=CARTESIAN_POINT('Ctrl Pts',(10.3990654189357,-23.6298416794532,5.74510895921686));
#16000=CARTESIAN_POINT('Ctrl Pts',(10.6133511332214,-22.3185580498516,8.4680174730597));
#16001=CARTESIAN_POINT('Ctrl Pts',(10.8276368475071,-19.9557065953293,10.3523286299233));
#16002=CARTESIAN_POINT('Ctrl Pts',(11.0419225617928,-17.592855140807,12.236639786787));
#16003=CARTESIAN_POINT('Ctrl Pts',(11.2562082760786,-14.6464275704035,12.9091426524948));
#16004=CARTESIAN_POINT('Ctrl Pts',(11.4704939903643,-11.7,13.5816455182026));
#16005=CARTESIAN_POINT('Ctrl Pts',(11.68477970465,-8.75357242959651,12.9091426524948));
#16006=CARTESIAN_POINT('Ctrl Pts',(11.8990654189357,-5.80714485919301,12.236639786787));
#16007=CARTESIAN_POINT('Ctrl Pts',(12.1133511332214,-3.4442934046707,10.3523286299233));
#16008=CARTESIAN_POINT('Ctrl Pts',(12.3276368475071,-1.08144195014836,8.4680174730597));
#16009=CARTESIAN_POINT('Ctrl Pts',(12.5419225617929,0.229841679453266,5.74510895921686));
#16010=CARTESIAN_POINT('Ctrl Pts',(12.7562082760786,1.5411253090549,3.02220044537403));
#16011=CARTESIAN_POINT('Ctrl Pts',(12.9704939903643,1.5411253090549,-2.08166817117217E-14));
#16012=CARTESIAN_POINT('Ctrl Pts',(13.18477970465,1.5411253090549,-3.02220044537405));
#16013=CARTESIAN_POINT('Ctrl Pts',(13.3990654189357,0.229841679453252,-5.74510895921687));
#16014=CARTESIAN_POINT('Ctrl Pts',(13.6133511332214,-1.08144195014838,-8.46801747305971));
#16015=CARTESIAN_POINT('Ctrl Pts',(13.8276368475071,-3.44429340467069,-10.3523286299233));
#16016=CARTESIAN_POINT('Ctrl Pts',(14.0419225617929,-5.80714485919301,-12.236639786787));
#16017=CARTESIAN_POINT('Ctrl Pts',(14.2562082760786,-8.75357242959651,-12.9091426524948));
#16018=CARTESIAN_POINT('Ctrl Pts',(14.4704939903643,-11.7,-13.5816455182026));
#16019=CARTESIAN_POINT('Ctrl Pts',(14.68477970465,-14.6464275704035,-12.9091426524948));
#16020=CARTESIAN_POINT('Ctrl Pts',(14.8990654189357,-17.592855140807,-12.236639786787));
#16021=CARTESIAN_POINT('Ctrl Pts',(15.1133511332214,-19.9557065953293,-10.3523286299233));
#16022=CARTESIAN_POINT('Ctrl Pts',(15.3276368475071,-22.3185580498516,-8.46801747305969));
#16023=CARTESIAN_POINT('Ctrl Pts',(15.5419225617929,-23.6298416794532,-5.74510895921687));
#16024=CARTESIAN_POINT('Ctrl Pts',(15.7562082760786,-24.9411253090549,-3.02220044537403));
#16025=CARTESIAN_POINT('Ctrl Pts',(15.9704939903643,-24.9411253090549,-6.93889390390723E-15));
#16026=CARTESIAN_POINT('Ctrl Pts',(16.18477970465,-24.9411253090549,3.02220044537403));
#16027=CARTESIAN_POINT('Ctrl Pts',(16.3990654189357,-23.6298416794532,5.74510895921686));
#16028=CARTESIAN_POINT('Ctrl Pts',(16.6133511332214,-22.3185580498516,8.46801747305969));
#16029=CARTESIAN_POINT('Ctrl Pts',(16.8276368475071,-19.9557065953293,10.3523286299233));
#16030=CARTESIAN_POINT('Ctrl Pts',(17.0419225617928,-17.592855140807,12.236639786787));
#16031=CARTESIAN_POINT('Ctrl Pts',(17.2562082760786,-14.6464275704035,12.9091426524948));
#16032=CARTESIAN_POINT('Ctrl Pts',(17.4704939903643,-11.7,13.5816455182026));
#16033=CARTESIAN_POINT('Ctrl Pts',(17.68477970465,-8.75357242959651,12.9091426524948));
#16034=CARTESIAN_POINT('Ctrl Pts',(17.8990654189357,-5.80714485919301,12.236639786787));
#16035=CARTESIAN_POINT('Ctrl Pts',(18.1133511332214,-3.4442934046707,10.3523286299233));
#16036=CARTESIAN_POINT('Ctrl Pts',(18.3276368475071,-1.08144195014837,8.46801747305969));
#16037=CARTESIAN_POINT('Ctrl Pts',(18.5419225617928,0.229841679453252,5.74510895921686));
#16038=CARTESIAN_POINT('Ctrl Pts',(18.7562082760786,1.5411253090549,3.02220044537405));
#16039=CARTESIAN_POINT('Ctrl Pts',(18.9704939903643,1.5411253090549,-1.38777878078145E-14));
#16040=CARTESIAN_POINT('Ctrl Pts',(19.18477970465,1.5411253090549,-3.02220044537404));
#16041=CARTESIAN_POINT('Ctrl Pts',(19.3990654189357,0.229841679453259,-5.74510895921686));
#16042=CARTESIAN_POINT('Ctrl Pts',(19.6133511332214,-1.08144195014838,-8.4680174730597));
#16043=CARTESIAN_POINT('Ctrl Pts',(19.8276368475071,-3.4442934046707,-10.3523286299233));
#16044=CARTESIAN_POINT('Ctrl Pts',(20.0419225617929,-5.80714485919302,-12.236639786787));
#16045=CARTESIAN_POINT('Ctrl Pts',(20.2562082760786,-8.75357242959651,-12.9091426524948));
#16046=CARTESIAN_POINT('Ctrl Pts',(20.4704939903643,-11.7,-13.5816455182026));
#16047=CARTESIAN_POINT('Ctrl Pts',(20.68477970465,-14.6464275704035,-12.9091426524948));
#16048=CARTESIAN_POINT('Ctrl Pts',(20.8990654189357,-17.592855140807,-12.236639786787));
#16049=CARTESIAN_POINT('Ctrl Pts',(21.1133511332214,-19.9557065953293,-10.3523286299233));
#16050=CARTESIAN_POINT('Ctrl Pts',(21.3276368475071,-22.3185580498516,-8.4680174730597));
#16051=CARTESIAN_POINT('Ctrl Pts',(21.5419225617929,-23.6298416794532,-5.74510895921687));
#16052=CARTESIAN_POINT('Ctrl Pts',(21.7562082760786,-24.9411253090549,-3.02220044537404));
#16053=CARTESIAN_POINT('Ctrl Pts',(21.9704939903643,-24.9411253090549,-3.46944695195361E-15));
#16054=CARTESIAN_POINT('Ctrl Pts',(22.18477970465,-24.9411253090549,3.02220044537403));
#16055=CARTESIAN_POINT('Ctrl Pts',(22.3990654189357,-23.6298416794532,5.74510895921686));
#16056=CARTESIAN_POINT('Ctrl Pts',(22.6133511332214,-22.3185580498516,8.46801747305969));
#16057=CARTESIAN_POINT('Ctrl Pts',(22.8276368475071,-19.9557065953293,10.3523286299233));
#16058=CARTESIAN_POINT('Ctrl Pts',(23.0419225617928,-17.592855140807,12.236639786787));
#16059=CARTESIAN_POINT('Ctrl Pts',(23.2562082760786,-14.6464275704035,12.9091426524948));
#16060=CARTESIAN_POINT('Ctrl Pts',(23.4704939903643,-11.7,13.5816455182026));
#16061=CARTESIAN_POINT('Ctrl Pts',(23.68477970465,-8.75357242959651,12.9091426524948));
#16062=CARTESIAN_POINT('Ctrl Pts',(23.8990654189357,-5.80714485919302,12.236639786787));
#16063=CARTESIAN_POINT('Ctrl Pts',(24.1133511332214,-3.4442934046707,10.3523286299233));
#16064=CARTESIAN_POINT('Ctrl Pts',(24.3276368475071,-1.08144195014837,8.46801747305969));
#16065=CARTESIAN_POINT('Ctrl Pts',(24.5419225617928,0.229841679453252,5.74510895921686));
#16066=CARTESIAN_POINT('Ctrl Pts',(24.7562082760786,1.5411253090549,3.02220044537404));
#16067=CARTESIAN_POINT('Ctrl Pts',(24.9704939903643,1.5411253090549,0.));
#16068=CARTESIAN_POINT('',(1.43524699518214,-0.329437345472555,-3.46944695195361E-15));
#16069=CARTESIAN_POINT('Origin',(-24.,2.30000000000001,3.46944695195361E-15));
#16070=CARTESIAN_POINT('',(-23.0295060096357,1.5411253090549,0.));
#16071=CARTESIAN_POINT('',(-22.5647530048179,-0.329437345472555,-6.93889390390723E-15));
#16072=CARTESIAN_POINT('',(-24.9704939903643,1.5411253090549,0.));
#16073=CARTESIAN_POINT('Origin',(-24.,1.3,-6.93889390390723E-15));
#16074=CARTESIAN_POINT('',(-25.4352469951821,-0.329437345472555,-1.38777878078145E-14));
#16075=CARTESIAN_POINT('Ctrl Pts',(-0.97049399036428,1.5411253090549,-6.93889390390723E-15));
#16076=CARTESIAN_POINT('Ctrl Pts',(-1.18477970465,1.5411253090549,3.02220044537404));
#16077=CARTESIAN_POINT('Ctrl Pts',(-1.39906541893571,0.229841679453259,
5.74510895921686));
#16078=CARTESIAN_POINT('Ctrl Pts',(-1.61335113322143,-1.08144195014837,
8.46801747305969));
#16079=CARTESIAN_POINT('Ctrl Pts',(-1.82763684750714,-3.4442934046707,10.3523286299233));
#16080=CARTESIAN_POINT('Ctrl Pts',(-2.04192256179286,-5.80714485919302,
12.236639786787));
#16081=CARTESIAN_POINT('Ctrl Pts',(-2.25620827607857,-8.75357242959651,
12.9091426524948));
#16082=CARTESIAN_POINT('Ctrl Pts',(-2.47049399036428,-11.7,13.5816455182026));
#16083=CARTESIAN_POINT('Ctrl Pts',(-2.68477970464999,-14.6464275704035,
12.9091426524948));
#16084=CARTESIAN_POINT('Ctrl Pts',(-2.89906541893571,-17.592855140807,12.236639786787));
#16085=CARTESIAN_POINT('Ctrl Pts',(-3.11335113322142,-19.9557065953293,
10.3523286299233));
#16086=CARTESIAN_POINT('Ctrl Pts',(-3.32763684750714,-22.3185580498516,
8.46801747305969));
#16087=CARTESIAN_POINT('Ctrl Pts',(-3.54192256179285,-23.6298416794532,
5.74510895921685));
#16088=CARTESIAN_POINT('Ctrl Pts',(-3.75620827607857,-24.9411253090549,
3.02220044537403));
#16089=CARTESIAN_POINT('Ctrl Pts',(-3.97049399036429,-24.9411253090549,
-6.93889390390723E-15));
#16090=CARTESIAN_POINT('Ctrl Pts',(-4.18477970464999,-24.9411253090549,
-3.02220044537404));
#16091=CARTESIAN_POINT('Ctrl Pts',(-4.39906541893571,-23.6298416794532,
-5.74510895921685));
#16092=CARTESIAN_POINT('Ctrl Pts',(-4.61335113322143,-22.3185580498516,
-8.46801747305969));
#16093=CARTESIAN_POINT('Ctrl Pts',(-4.82763684750714,-19.9557065953293,
-10.3523286299233));
#16094=CARTESIAN_POINT('Ctrl Pts',(-5.04192256179286,-17.592855140807,-12.236639786787));
#16095=CARTESIAN_POINT('Ctrl Pts',(-5.25620827607857,-14.6464275704035,
-12.9091426524948));
#16096=CARTESIAN_POINT('Ctrl Pts',(-5.47049399036429,-11.7,-13.5816455182026));
#16097=CARTESIAN_POINT('Ctrl Pts',(-5.68477970464999,-8.75357242959651,
-12.9091426524948));
#16098=CARTESIAN_POINT('Ctrl Pts',(-5.89906541893571,-5.80714485919302,
-12.236639786787));
#16099=CARTESIAN_POINT('Ctrl Pts',(-6.11335113322142,-3.4442934046707,-10.3523286299233));
#16100=CARTESIAN_POINT('Ctrl Pts',(-6.32763684750714,-1.08144195014838,
-8.46801747305971));
#16101=CARTESIAN_POINT('Ctrl Pts',(-6.54192256179285,0.229841679453252,
-5.74510895921688));
#16102=CARTESIAN_POINT('Ctrl Pts',(-6.75620827607857,1.5411253090549,-3.02220044537405));
#16103=CARTESIAN_POINT('Ctrl Pts',(-6.97049399036428,1.54112530905488,-6.93889390390723E-15));
#16104=CARTESIAN_POINT('Ctrl Pts',(-7.18477970465,1.5411253090549,3.02220044537401));
#16105=CARTESIAN_POINT('Ctrl Pts',(-7.39906541893571,0.229841679453252,
5.74510895921687));
#16106=CARTESIAN_POINT('Ctrl Pts',(-7.61335113322142,-1.08144195014837,
8.4680174730597));
#16107=CARTESIAN_POINT('Ctrl Pts',(-7.82763684750714,-3.4442934046707,10.3523286299233));
#16108=CARTESIAN_POINT('Ctrl Pts',(-8.04192256179286,-5.80714485919302,
12.236639786787));
#16109=CARTESIAN_POINT('Ctrl Pts',(-8.25620827607856,-8.75357242959651,
12.9091426524948));
#16110=CARTESIAN_POINT('Ctrl Pts',(-8.47049399036428,-11.7,13.5816455182026));
#16111=CARTESIAN_POINT('Ctrl Pts',(-8.68477970464999,-14.6464275704035,
12.9091426524948));
#16112=CARTESIAN_POINT('Ctrl Pts',(-8.89906541893571,-17.592855140807,12.236639786787));
#16113=CARTESIAN_POINT('Ctrl Pts',(-9.11335113322142,-19.9557065953293,
10.3523286299233));
#16114=CARTESIAN_POINT('Ctrl Pts',(-9.32763684750714,-22.3185580498516,
8.4680174730597));
#16115=CARTESIAN_POINT('Ctrl Pts',(-9.54192256179285,-23.6298416794532,
5.74510895921686));
#16116=CARTESIAN_POINT('Ctrl Pts',(-9.75620827607857,-24.9411253090549,
3.02220044537403));
#16117=CARTESIAN_POINT('Ctrl Pts',(-9.97049399036428,-24.9411253090549,
-6.93889390390723E-15));
#16118=CARTESIAN_POINT('Ctrl Pts',(-10.18477970465,-24.9411253090549,-3.02220044537404));
#16119=CARTESIAN_POINT('Ctrl Pts',(-10.3990654189357,-23.6298416794532,
-5.74510895921686));
#16120=CARTESIAN_POINT('Ctrl Pts',(-10.6133511332214,-22.3185580498516,
-8.46801747305971));
#16121=CARTESIAN_POINT('Ctrl Pts',(-10.8276368475071,-19.9557065953293,
-10.3523286299233));
#16122=CARTESIAN_POINT('Ctrl Pts',(-11.0419225617928,-17.5928551408069,
-12.236639786787));
#16123=CARTESIAN_POINT('Ctrl Pts',(-11.2562082760786,-14.6464275704035,
-12.9091426524948));
#16124=CARTESIAN_POINT('Ctrl Pts',(-11.4704939903643,-11.7,-13.5816455182026));
#16125=CARTESIAN_POINT('Ctrl Pts',(-11.68477970465,-8.75357242959649,-12.9091426524948));
#16126=CARTESIAN_POINT('Ctrl Pts',(-11.8990654189357,-5.80714485919302,
-12.236639786787));
#16127=CARTESIAN_POINT('Ctrl Pts',(-12.1133511332214,-3.44429340467069,
-10.3523286299234));
#16128=CARTESIAN_POINT('Ctrl Pts',(-12.3276368475071,-1.08144195014838,
-8.46801747305969));
#16129=CARTESIAN_POINT('Ctrl Pts',(-12.5419225617929,0.229841679453252,
-5.74510895921687));
#16130=CARTESIAN_POINT('Ctrl Pts',(-12.7562082760786,1.54112530905491,-3.02220044537405));
#16131=CARTESIAN_POINT('Ctrl Pts',(-12.9704939903643,1.5411253090549,0.));
#16132=CARTESIAN_POINT('Ctrl Pts',(-13.18477970465,1.5411253090549,3.02220044537401));
#16133=CARTESIAN_POINT('Ctrl Pts',(-13.3990654189357,0.229841679453252,
5.74510895921686));
#16134=CARTESIAN_POINT('Ctrl Pts',(-13.6133511332214,-1.08144195014837,
8.46801747305969));
#16135=CARTESIAN_POINT('Ctrl Pts',(-13.8276368475071,-3.4442934046707,10.3523286299233));
#16136=CARTESIAN_POINT('Ctrl Pts',(-14.0419225617929,-5.80714485919302,
12.236639786787));
#16137=CARTESIAN_POINT('Ctrl Pts',(-14.2562082760786,-8.75357242959651,
12.9091426524948));
#16138=CARTESIAN_POINT('Ctrl Pts',(-14.4704939903643,-11.7,13.5816455182026));
#16139=CARTESIAN_POINT('Ctrl Pts',(-14.68477970465,-14.6464275704035,12.9091426524948));
#16140=CARTESIAN_POINT('Ctrl Pts',(-14.8990654189357,-17.5928551408069,
12.236639786787));
#16141=CARTESIAN_POINT('Ctrl Pts',(-15.1133511332214,-19.9557065953293,
10.3523286299233));
#16142=CARTESIAN_POINT('Ctrl Pts',(-15.3276368475071,-22.3185580498516,
8.46801747305968));
#16143=CARTESIAN_POINT('Ctrl Pts',(-15.5419225617929,-23.6298416794532,
5.74510895921686));
#16144=CARTESIAN_POINT('Ctrl Pts',(-15.7562082760786,-24.9411253090549,
3.02220044537403));
#16145=CARTESIAN_POINT('Ctrl Pts',(-15.9704939903643,-24.9411253090549,
0.));
#16146=CARTESIAN_POINT('Ctrl Pts',(-16.18477970465,-24.9411253090549,-3.02220044537402));
#16147=CARTESIAN_POINT('Ctrl Pts',(-16.3990654189357,-23.6298416794532,
-5.74510895921687));
#16148=CARTESIAN_POINT('Ctrl Pts',(-16.6133511332214,-22.3185580498516,
-8.4680174730597));
#16149=CARTESIAN_POINT('Ctrl Pts',(-16.8276368475071,-19.9557065953293,
-10.3523286299233));
#16150=CARTESIAN_POINT('Ctrl Pts',(-17.0419225617929,-17.5928551408069,
-12.236639786787));
#16151=CARTESIAN_POINT('Ctrl Pts',(-17.2562082760786,-14.6464275704035,
-12.9091426524948));
#16152=CARTESIAN_POINT('Ctrl Pts',(-17.4704939903643,-11.7,-13.5816455182026));
#16153=CARTESIAN_POINT('Ctrl Pts',(-17.68477970465,-8.75357242959651,-12.9091426524948));
#16154=CARTESIAN_POINT('Ctrl Pts',(-17.8990654189357,-5.80714485919301,
-12.236639786787));
#16155=CARTESIAN_POINT('Ctrl Pts',(-18.1133511332214,-3.4442934046707,-10.3523286299233));
#16156=CARTESIAN_POINT('Ctrl Pts',(-18.3276368475072,-1.08144195014838,
-8.46801747305968));
#16157=CARTESIAN_POINT('Ctrl Pts',(-18.5419225617929,0.229841679453252,
-5.74510895921686));
#16158=CARTESIAN_POINT('Ctrl Pts',(-18.7562082760786,1.5411253090549,-3.02220044537404));
#16159=CARTESIAN_POINT('Ctrl Pts',(-18.9704939903643,1.5411253090549,-3.46944695195361E-15));
#16160=CARTESIAN_POINT('Ctrl Pts',(-19.18477970465,1.5411253090549,3.02220044537403));
#16161=CARTESIAN_POINT('Ctrl Pts',(-19.3990654189357,0.229841679453252,
5.74510895921686));
#16162=CARTESIAN_POINT('Ctrl Pts',(-19.6133511332214,-1.08144195014837,
8.4680174730597));
#16163=CARTESIAN_POINT('Ctrl Pts',(-19.8276368475071,-3.4442934046707,10.3523286299233));
#16164=CARTESIAN_POINT('Ctrl Pts',(-20.0419225617929,-5.80714485919302,
12.236639786787));
#16165=CARTESIAN_POINT('Ctrl Pts',(-20.2562082760786,-8.75357242959651,
12.9091426524948));
#16166=CARTESIAN_POINT('Ctrl Pts',(-20.4704939903643,-11.7,13.5816455182026));
#16167=CARTESIAN_POINT('Ctrl Pts',(-20.68477970465,-14.6464275704035,12.9091426524948));
#16168=CARTESIAN_POINT('Ctrl Pts',(-20.8990654189357,-17.5928551408069,
12.236639786787));
#16169=CARTESIAN_POINT('Ctrl Pts',(-21.1133511332214,-19.9557065953293,
10.3523286299233));
#16170=CARTESIAN_POINT('Ctrl Pts',(-21.3276368475072,-22.3185580498516,
8.4680174730597));
#16171=CARTESIAN_POINT('Ctrl Pts',(-21.5419225617929,-23.6298416794532,
5.74510895921686));
#16172=CARTESIAN_POINT('Ctrl Pts',(-21.7562082760786,-24.9411253090549,
3.02220044537405));
#16173=CARTESIAN_POINT('Ctrl Pts',(-21.9704939903643,-24.9411253090549,
3.46944695195361E-15));
#16174=CARTESIAN_POINT('Ctrl Pts',(-22.18477970465,-24.9411253090549,-3.02220044537404));
#16175=CARTESIAN_POINT('Ctrl Pts',(-22.3990654189357,-23.6298416794532,
-5.74510895921686));
#16176=CARTESIAN_POINT('Ctrl Pts',(-22.6133511332214,-22.3185580498516,
-8.4680174730597));
#16177=CARTESIAN_POINT('Ctrl Pts',(-22.8276368475072,-19.9557065953293,
-10.3523286299233));
#16178=CARTESIAN_POINT('Ctrl Pts',(-23.0419225617929,-17.592855140807,-12.236639786787));
#16179=CARTESIAN_POINT('Ctrl Pts',(-23.2562082760786,-14.6464275704035,
-12.9091426524948));
#16180=CARTESIAN_POINT('Ctrl Pts',(-23.4704939903643,-11.7,-13.5816455182026));
#16181=CARTESIAN_POINT('Ctrl Pts',(-23.68477970465,-8.75357242959651,-12.9091426524948));
#16182=CARTESIAN_POINT('Ctrl Pts',(-23.8990654189357,-5.80714485919301,
-12.236639786787));
#16183=CARTESIAN_POINT('Ctrl Pts',(-24.1133511332214,-3.4442934046707,-10.3523286299233));
#16184=CARTESIAN_POINT('Ctrl Pts',(-24.3276368475071,-1.08144195014838,
-8.46801747305971));
#16185=CARTESIAN_POINT('Ctrl Pts',(-24.5419225617929,0.229841679453259,
-5.74510895921687));
#16186=CARTESIAN_POINT('Ctrl Pts',(-24.7562082760786,1.54112530905491,-3.02220044537405));
#16187=CARTESIAN_POINT('Ctrl Pts',(-24.9704939903643,1.5411253090549,0.));
#16188=CARTESIAN_POINT('Ctrl Pts',(-1.9,-2.2,0.));
#16189=CARTESIAN_POINT('Ctrl Pts',(-2.11428571428572,-2.19999999999999,
2.16831300670641));
#16190=CARTESIAN_POINT('Ctrl Pts',(-2.32857142857143,-3.14079575492701,
4.1218955216168));
#16191=CARTESIAN_POINT('Ctrl Pts',(-2.54285714285714,-4.08159150985402,
6.07547803652717));
#16192=CARTESIAN_POINT('Ctrl Pts',(-2.75714285714286,-5.77684688234203,
7.42739908344627));
#16193=CARTESIAN_POINT('Ctrl Pts',(-2.97142857142857,-7.47210225483002,
8.77932013036537));
#16194=CARTESIAN_POINT('Ctrl Pts',(-3.18571428571429,-9.58605112741499,
9.2618151657273));
#16195=CARTESIAN_POINT('Ctrl Pts',(-3.4,-11.7,9.74431020108924));
#16196=CARTESIAN_POINT('Ctrl Pts',(-3.61428571428572,-13.813948872585,9.26181516572731));
#16197=CARTESIAN_POINT('Ctrl Pts',(-3.82857142857143,-15.92789774517,8.77932013036537));
#16198=CARTESIAN_POINT('Ctrl Pts',(-4.04285714285715,-17.623153117658,7.42739908344628));
#16199=CARTESIAN_POINT('Ctrl Pts',(-4.25714285714286,-19.318408490146,6.07547803652718));
#16200=CARTESIAN_POINT('Ctrl Pts',(-4.47142857142857,-20.259204245073,4.1218955216168));
#16201=CARTESIAN_POINT('Ctrl Pts',(-4.68571428571429,-21.2,2.16831300670642));
#16202=CARTESIAN_POINT('Ctrl Pts',(-4.9,-21.2,-1.04083408558608E-14));
#16203=CARTESIAN_POINT('Ctrl Pts',(-5.11428571428572,-21.2,-2.16831300670643));
#16204=CARTESIAN_POINT('Ctrl Pts',(-5.32857142857143,-20.259204245073,-4.1218955216168));
#16205=CARTESIAN_POINT('Ctrl Pts',(-5.54285714285714,-19.318408490146,-6.07547803652718));
#16206=CARTESIAN_POINT('Ctrl Pts',(-5.75714285714286,-17.623153117658,-7.42739908344628));
#16207=CARTESIAN_POINT('Ctrl Pts',(-5.97142857142858,-15.92789774517,-8.7793201303654));
#16208=CARTESIAN_POINT('Ctrl Pts',(-6.18571428571429,-13.813948872585,-9.26181516572732));
#16209=CARTESIAN_POINT('Ctrl Pts',(-6.4,-11.7,-9.74431020108927));
#16210=CARTESIAN_POINT('Ctrl Pts',(-6.61428571428572,-9.58605112741499,
-9.26181516572733));
#16211=CARTESIAN_POINT('Ctrl Pts',(-6.82857142857144,-7.47210225483002,
-8.77932013036538));
#16212=CARTESIAN_POINT('Ctrl Pts',(-7.04285714285714,-5.77684688234203,
-7.42739908344628));
#16213=CARTESIAN_POINT('Ctrl Pts',(-7.25714285714286,-4.08159150985404,
-6.07547803652718));
#16214=CARTESIAN_POINT('Ctrl Pts',(-7.47142857142857,-3.14079575492701,
-4.12189552161681));
#16215=CARTESIAN_POINT('Ctrl Pts',(-7.68571428571429,-2.2,-2.16831300670643));
#16216=CARTESIAN_POINT('Ctrl Pts',(-7.9,-2.2,-3.46944695195361E-15));
#16217=CARTESIAN_POINT('Ctrl Pts',(-8.11428571428572,-2.20000000000001,
2.16831300670642));
#16218=CARTESIAN_POINT('Ctrl Pts',(-8.32857142857143,-3.14079575492702,
4.12189552161678));
#16219=CARTESIAN_POINT('Ctrl Pts',(-8.54285714285714,-4.08159150985404,
6.07547803652716));
#16220=CARTESIAN_POINT('Ctrl Pts',(-8.75714285714286,-5.77684688234202,
7.42739908344627));
#16221=CARTESIAN_POINT('Ctrl Pts',(-8.97142857142857,-7.47210225483001,
8.77932013036537));
#16222=CARTESIAN_POINT('Ctrl Pts',(-9.18571428571429,-9.58605112741501,
9.26181516572731));
#16223=CARTESIAN_POINT('Ctrl Pts',(-9.4,-11.7,9.74431020108925));
#16224=CARTESIAN_POINT('Ctrl Pts',(-9.61428571428571,-13.813948872585,9.26181516572731));
#16225=CARTESIAN_POINT('Ctrl Pts',(-9.82857142857143,-15.92789774517,8.77932013036538));
#16226=CARTESIAN_POINT('Ctrl Pts',(-10.0428571428572,-17.6231531176579,
7.42739908344626));
#16227=CARTESIAN_POINT('Ctrl Pts',(-10.2571428571429,-19.3184084901459,
6.07547803652716));
#16228=CARTESIAN_POINT('Ctrl Pts',(-10.4714285714286,-20.259204245073,4.12189552161679));
#16229=CARTESIAN_POINT('Ctrl Pts',(-10.6857142857143,-21.2,2.16831300670642));
#16230=CARTESIAN_POINT('Ctrl Pts',(-10.9,-21.2,-6.93889390390723E-15));
#16231=CARTESIAN_POINT('Ctrl Pts',(-11.1142857142857,-21.2,-2.16831300670643));
#16232=CARTESIAN_POINT('Ctrl Pts',(-11.3285714285714,-20.259204245073,-4.12189552161681));
#16233=CARTESIAN_POINT('Ctrl Pts',(-11.5428571428571,-19.3184084901459,
-6.07547803652717));
#16234=CARTESIAN_POINT('Ctrl Pts',(-11.7571428571429,-17.623153117658,-7.42739908344627));
#16235=CARTESIAN_POINT('Ctrl Pts',(-11.9714285714286,-15.92789774517,-8.77932013036536));
#16236=CARTESIAN_POINT('Ctrl Pts',(-12.1857142857143,-13.813948872585,-9.26181516572733));
#16237=CARTESIAN_POINT('Ctrl Pts',(-12.4,-11.7,-9.74431020108925));
#16238=CARTESIAN_POINT('Ctrl Pts',(-12.6142857142857,-9.58605112741501,
-9.26181516572733));
#16239=CARTESIAN_POINT('Ctrl Pts',(-12.8285714285714,-7.47210225483001,
-8.77932013036539));
#16240=CARTESIAN_POINT('Ctrl Pts',(-13.0428571428571,-5.77684688234202,
-7.4273990834463));
#16241=CARTESIAN_POINT('Ctrl Pts',(-13.2571428571429,-4.08159150985404,
-6.07547803652718));
#16242=CARTESIAN_POINT('Ctrl Pts',(-13.4714285714286,-3.14079575492702,
-4.12189552161681));
#16243=CARTESIAN_POINT('Ctrl Pts',(-13.6857142857143,-2.2,-2.16831300670643));
#16244=CARTESIAN_POINT('Ctrl Pts',(-13.9,-2.2,0.));
#16245=CARTESIAN_POINT('Ctrl Pts',(-14.1142857142857,-2.19999999999999,
2.16831300670641));
#16246=CARTESIAN_POINT('Ctrl Pts',(-14.3285714285714,-3.14079575492702,
4.1218955216168));
#16247=CARTESIAN_POINT('Ctrl Pts',(-14.5428571428571,-4.08159150985404,
6.07547803652717));
#16248=CARTESIAN_POINT('Ctrl Pts',(-14.7571428571429,-5.77684688234203,
7.42739908344626));
#16249=CARTESIAN_POINT('Ctrl Pts',(-14.9714285714286,-7.47210225483001,
8.77932013036538));
#16250=CARTESIAN_POINT('Ctrl Pts',(-15.1857142857143,-9.58605112741501,
9.26181516572731));
#16251=CARTESIAN_POINT('Ctrl Pts',(-15.4,-11.7,9.74431020108925));
#16252=CARTESIAN_POINT('Ctrl Pts',(-15.6142857142857,-13.813948872585,9.26181516572731));
#16253=CARTESIAN_POINT('Ctrl Pts',(-15.8285714285714,-15.92789774517,8.77932013036537));
#16254=CARTESIAN_POINT('Ctrl Pts',(-16.0428571428571,-17.6231531176579,
7.42739908344627));
#16255=CARTESIAN_POINT('Ctrl Pts',(-16.2571428571429,-19.3184084901459,
6.07547803652717));
#16256=CARTESIAN_POINT('Ctrl Pts',(-16.4714285714286,-20.259204245073,4.12189552161679));
#16257=CARTESIAN_POINT('Ctrl Pts',(-16.6857142857143,-21.2,2.16831300670642));
#16258=CARTESIAN_POINT('Ctrl Pts',(-16.9,-21.2,-6.93889390390723E-15));
#16259=CARTESIAN_POINT('Ctrl Pts',(-17.1142857142857,-21.2,-2.16831300670643));
#16260=CARTESIAN_POINT('Ctrl Pts',(-17.3285714285715,-20.259204245073,-4.1218955216168));
#16261=CARTESIAN_POINT('Ctrl Pts',(-17.5428571428572,-19.3184084901459,
-6.07547803652717));
#16262=CARTESIAN_POINT('Ctrl Pts',(-17.7571428571429,-17.623153117658,-7.42739908344627));
#16263=CARTESIAN_POINT('Ctrl Pts',(-17.9714285714286,-15.92789774517,-8.77932013036538));
#16264=CARTESIAN_POINT('Ctrl Pts',(-18.1857142857143,-13.813948872585,-9.26181516572732));
#16265=CARTESIAN_POINT('Ctrl Pts',(-18.4,-11.7,-9.74431020108925));
#16266=CARTESIAN_POINT('Ctrl Pts',(-18.6142857142857,-9.58605112741501,
-9.26181516572731));
#16267=CARTESIAN_POINT('Ctrl Pts',(-18.8285714285714,-7.47210225483001,
-8.77932013036538));
#16268=CARTESIAN_POINT('Ctrl Pts',(-19.0428571428572,-5.77684688234203,
-7.42739908344629));
#16269=CARTESIAN_POINT('Ctrl Pts',(-19.2571428571429,-4.08159150985404,
-6.07547803652718));
#16270=CARTESIAN_POINT('Ctrl Pts',(-19.4714285714286,-3.14079575492701,
-4.1218955216168));
#16271=CARTESIAN_POINT('Ctrl Pts',(-19.6857142857143,-2.2,-2.16831300670644));
#16272=CARTESIAN_POINT('Ctrl Pts',(-19.9,-2.2,-3.46944695195361E-15));
#16273=CARTESIAN_POINT('Ctrl Pts',(-20.1142857142857,-2.19999999999999,
2.16831300670643));
#16274=CARTESIAN_POINT('Ctrl Pts',(-20.3285714285714,-3.14079575492702,
4.1218955216168));
#16275=CARTESIAN_POINT('Ctrl Pts',(-20.5428571428571,-4.08159150985404,
6.07547803652716));
#16276=CARTESIAN_POINT('Ctrl Pts',(-20.7571428571429,-5.77684688234202,
7.42739908344627));
#16277=CARTESIAN_POINT('Ctrl Pts',(-20.9714285714286,-7.47210225483001,
8.77932013036537));
#16278=CARTESIAN_POINT('Ctrl Pts',(-21.1857142857143,-9.58605112741501,
9.2618151657273));
#16279=CARTESIAN_POINT('Ctrl Pts',(-21.4,-11.7,9.74431020108925));
#16280=CARTESIAN_POINT('Ctrl Pts',(-21.6142857142857,-13.813948872585,9.26181516572731));
#16281=CARTESIAN_POINT('Ctrl Pts',(-21.8285714285714,-15.92789774517,8.77932013036537));
#16282=CARTESIAN_POINT('Ctrl Pts',(-22.0428571428571,-17.6231531176579,
7.42739908344627));
#16283=CARTESIAN_POINT('Ctrl Pts',(-22.2571428571429,-19.3184084901459,
6.07547803652717));
#16284=CARTESIAN_POINT('Ctrl Pts',(-22.4714285714286,-20.259204245073,4.1218955216168));
#16285=CARTESIAN_POINT('Ctrl Pts',(-22.6857142857143,-21.2,2.16831300670641));
#16286=CARTESIAN_POINT('Ctrl Pts',(-22.9,-21.2,-6.93889390390723E-15));
#16287=CARTESIAN_POINT('Ctrl Pts',(-23.1142857142857,-21.2,-2.16831300670642));
#16288=CARTESIAN_POINT('Ctrl Pts',(-23.3285714285715,-20.259204245073,-4.1218955216168));
#16289=CARTESIAN_POINT('Ctrl Pts',(-23.5428571428572,-19.318408490146,-6.07547803652718));
#16290=CARTESIAN_POINT('Ctrl Pts',(-23.7571428571429,-17.623153117658,-7.42739908344627));
#16291=CARTESIAN_POINT('Ctrl Pts',(-23.9714285714286,-15.9278977451699,
-8.77932013036538));
#16292=CARTESIAN_POINT('Ctrl Pts',(-24.1857142857143,-13.813948872585,-9.26181516572731));
#16293=CARTESIAN_POINT('Ctrl Pts',(-24.4,-11.7,-9.74431020108925));
#16294=CARTESIAN_POINT('Ctrl Pts',(-24.6142857142857,-9.58605112741501,
-9.26181516572732));
#16295=CARTESIAN_POINT('Ctrl Pts',(-24.8285714285714,-7.47210225483001,
-8.77932013036537));
#16296=CARTESIAN_POINT('Ctrl Pts',(-25.0428571428572,-5.77684688234203,
-7.42739908344628));
#16297=CARTESIAN_POINT('Ctrl Pts',(-25.2571428571429,-4.08159150985402,
-6.07547803652718));
#16298=CARTESIAN_POINT('Ctrl Pts',(-25.4714285714286,-3.14079575492701,
-4.12189552161682));
#16299=CARTESIAN_POINT('Ctrl Pts',(-25.6857142857143,-2.20000000000001,
-2.16831300670643));
#16300=CARTESIAN_POINT('Ctrl Pts',(-25.9,-2.20000000000001,-1.38777878078145E-14));
#16301=CARTESIAN_POINT('Ctrl Pts',(-0.97049399036428,1.5411253090549,-6.93889390390723E-15));
#16302=CARTESIAN_POINT('Ctrl Pts',(-1.18477970465,1.5411253090549,3.02220044537404));
#16303=CARTESIAN_POINT('Ctrl Pts',(-1.39906541893571,0.229841679453259,
5.74510895921686));
#16304=CARTESIAN_POINT('Ctrl Pts',(-1.61335113322143,-1.08144195014837,
8.46801747305969));
#16305=CARTESIAN_POINT('Ctrl Pts',(-1.82763684750714,-3.4442934046707,10.3523286299233));
#16306=CARTESIAN_POINT('Ctrl Pts',(-2.04192256179285,-5.80714485919302,
12.236639786787));
#16307=CARTESIAN_POINT('Ctrl Pts',(-2.25620827607857,-8.75357242959651,
12.9091426524948));
#16308=CARTESIAN_POINT('Ctrl Pts',(-2.47049399036428,-11.7,13.5816455182026));
#16309=CARTESIAN_POINT('Ctrl Pts',(-2.68477970464999,-14.6464275704035,
12.9091426524948));
#16310=CARTESIAN_POINT('Ctrl Pts',(-2.89906541893571,-17.592855140807,12.236639786787));
#16311=CARTESIAN_POINT('Ctrl Pts',(-3.11335113322142,-19.9557065953293,
10.3523286299233));
#16312=CARTESIAN_POINT('Ctrl Pts',(-3.32763684750714,-22.3185580498516,
8.46801747305969));
#16313=CARTESIAN_POINT('Ctrl Pts',(-3.54192256179285,-23.6298416794532,
5.74510895921685));
#16314=CARTESIAN_POINT('Ctrl Pts',(-3.75620827607857,-24.9411253090549,
3.02220044537403));
#16315=CARTESIAN_POINT('Ctrl Pts',(-3.97049399036428,-24.9411253090549,
-6.93889390390723E-15));
#16316=CARTESIAN_POINT('Ctrl Pts',(-4.18477970464999,-24.9411253090549,
-3.02220044537404));
#16317=CARTESIAN_POINT('Ctrl Pts',(-4.39906541893571,-23.6298416794532,
-5.74510895921685));
#16318=CARTESIAN_POINT('Ctrl Pts',(-4.61335113322142,-22.3185580498516,
-8.46801747305969));
#16319=CARTESIAN_POINT('Ctrl Pts',(-4.82763684750714,-19.9557065953293,
-10.3523286299233));
#16320=CARTESIAN_POINT('Ctrl Pts',(-5.04192256179286,-17.592855140807,-12.236639786787));
#16321=CARTESIAN_POINT('Ctrl Pts',(-5.25620827607857,-14.6464275704035,
-12.9091426524948));
#16322=CARTESIAN_POINT('Ctrl Pts',(-5.47049399036429,-11.7,-13.5816455182026));
#16323=CARTESIAN_POINT('Ctrl Pts',(-5.68477970464999,-8.75357242959651,
-12.9091426524948));
#16324=CARTESIAN_POINT('Ctrl Pts',(-5.89906541893571,-5.80714485919302,
-12.236639786787));
#16325=CARTESIAN_POINT('Ctrl Pts',(-6.11335113322142,-3.4442934046707,-10.3523286299233));
#16326=CARTESIAN_POINT('Ctrl Pts',(-6.32763684750714,-1.08144195014838,
-8.46801747305971));
#16327=CARTESIAN_POINT('Ctrl Pts',(-6.54192256179285,0.229841679453252,
-5.74510895921688));
#16328=CARTESIAN_POINT('Ctrl Pts',(-6.75620827607857,1.5411253090549,-3.02220044537405));
#16329=CARTESIAN_POINT('Ctrl Pts',(-6.97049399036428,1.54112530905488,-6.93889390390723E-15));
#16330=CARTESIAN_POINT('Ctrl Pts',(-7.18477970465,1.5411253090549,3.02220044537401));
#16331=CARTESIAN_POINT('Ctrl Pts',(-7.39906541893571,0.229841679453252,
5.74510895921687));
#16332=CARTESIAN_POINT('Ctrl Pts',(-7.61335113322143,-1.08144195014837,
8.4680174730597));
#16333=CARTESIAN_POINT('Ctrl Pts',(-7.82763684750714,-3.4442934046707,10.3523286299233));
#16334=CARTESIAN_POINT('Ctrl Pts',(-8.04192256179286,-5.80714485919302,
12.236639786787));
#16335=CARTESIAN_POINT('Ctrl Pts',(-8.25620827607856,-8.75357242959651,
12.9091426524948));
#16336=CARTESIAN_POINT('Ctrl Pts',(-8.47049399036428,-11.7,13.5816455182026));
#16337=CARTESIAN_POINT('Ctrl Pts',(-8.68477970464999,-14.6464275704035,
12.9091426524948));
#16338=CARTESIAN_POINT('Ctrl Pts',(-8.89906541893571,-17.592855140807,12.236639786787));
#16339=CARTESIAN_POINT('Ctrl Pts',(-9.11335113322142,-19.9557065953293,
10.3523286299233));
#16340=CARTESIAN_POINT('Ctrl Pts',(-9.32763684750714,-22.3185580498516,
8.4680174730597));
#16341=CARTESIAN_POINT('Ctrl Pts',(-9.54192256179285,-23.6298416794532,
5.74510895921686));
#16342=CARTESIAN_POINT('Ctrl Pts',(-9.75620827607857,-24.9411253090549,
3.02220044537403));
#16343=CARTESIAN_POINT('Ctrl Pts',(-9.97049399036428,-24.9411253090549,
-6.93889390390723E-15));
#16344=CARTESIAN_POINT('Ctrl Pts',(-10.18477970465,-24.9411253090549,-3.02220044537404));
#16345=CARTESIAN_POINT('Ctrl Pts',(-10.3990654189357,-23.6298416794532,
-5.74510895921686));
#16346=CARTESIAN_POINT('Ctrl Pts',(-10.6133511332214,-22.3185580498516,
-8.46801747305971));
#16347=CARTESIAN_POINT('Ctrl Pts',(-10.8276368475071,-19.9557065953293,
-10.3523286299233));
#16348=CARTESIAN_POINT('Ctrl Pts',(-11.0419225617928,-17.5928551408069,
-12.236639786787));
#16349=CARTESIAN_POINT('Ctrl Pts',(-11.2562082760786,-14.6464275704035,
-12.9091426524948));
#16350=CARTESIAN_POINT('Ctrl Pts',(-11.4704939903643,-11.7,-13.5816455182026));
#16351=CARTESIAN_POINT('Ctrl Pts',(-11.68477970465,-8.75357242959649,-12.9091426524948));
#16352=CARTESIAN_POINT('Ctrl Pts',(-11.8990654189357,-5.80714485919302,
-12.236639786787));
#16353=CARTESIAN_POINT('Ctrl Pts',(-12.1133511332214,-3.44429340467069,
-10.3523286299234));
#16354=CARTESIAN_POINT('Ctrl Pts',(-12.3276368475071,-1.08144195014838,
-8.46801747305969));
#16355=CARTESIAN_POINT('Ctrl Pts',(-12.5419225617929,0.229841679453252,
-5.74510895921687));
#16356=CARTESIAN_POINT('Ctrl Pts',(-12.7562082760786,1.54112530905491,-3.02220044537405));
#16357=CARTESIAN_POINT('Ctrl Pts',(-12.9704939903643,1.5411253090549,0.));
#16358=CARTESIAN_POINT('Ctrl Pts',(-13.18477970465,1.5411253090549,3.02220044537401));
#16359=CARTESIAN_POINT('Ctrl Pts',(-13.3990654189357,0.229841679453252,
5.74510895921686));
#16360=CARTESIAN_POINT('Ctrl Pts',(-13.6133511332214,-1.08144195014837,
8.46801747305969));
#16361=CARTESIAN_POINT('Ctrl Pts',(-13.8276368475071,-3.4442934046707,10.3523286299233));
#16362=CARTESIAN_POINT('Ctrl Pts',(-14.0419225617929,-5.80714485919302,
12.236639786787));
#16363=CARTESIAN_POINT('Ctrl Pts',(-14.2562082760786,-8.75357242959651,
12.9091426524948));
#16364=CARTESIAN_POINT('Ctrl Pts',(-14.4704939903643,-11.7,13.5816455182026));
#16365=CARTESIAN_POINT('Ctrl Pts',(-14.68477970465,-14.6464275704035,12.9091426524948));
#16366=CARTESIAN_POINT('Ctrl Pts',(-14.8990654189357,-17.5928551408069,
12.236639786787));
#16367=CARTESIAN_POINT('Ctrl Pts',(-15.1133511332214,-19.9557065953293,
10.3523286299233));
#16368=CARTESIAN_POINT('Ctrl Pts',(-15.3276368475071,-22.3185580498516,
8.46801747305968));
#16369=CARTESIAN_POINT('Ctrl Pts',(-15.5419225617929,-23.6298416794532,
5.74510895921686));
#16370=CARTESIAN_POINT('Ctrl Pts',(-15.7562082760786,-24.9411253090549,
3.02220044537403));
#16371=CARTESIAN_POINT('Ctrl Pts',(-15.9704939903643,-24.9411253090549,
0.));
#16372=CARTESIAN_POINT('Ctrl Pts',(-16.18477970465,-24.9411253090549,-3.02220044537402));
#16373=CARTESIAN_POINT('Ctrl Pts',(-16.3990654189357,-23.6298416794532,
-5.74510895921687));
#16374=CARTESIAN_POINT('Ctrl Pts',(-16.6133511332214,-22.3185580498516,
-8.4680174730597));
#16375=CARTESIAN_POINT('Ctrl Pts',(-16.8276368475071,-19.9557065953293,
-10.3523286299233));
#16376=CARTESIAN_POINT('Ctrl Pts',(-17.0419225617929,-17.5928551408069,
-12.236639786787));
#16377=CARTESIAN_POINT('Ctrl Pts',(-17.2562082760786,-14.6464275704035,
-12.9091426524948));
#16378=CARTESIAN_POINT('Ctrl Pts',(-17.4704939903643,-11.7,-13.5816455182026));
#16379=CARTESIAN_POINT('Ctrl Pts',(-17.68477970465,-8.75357242959651,-12.9091426524948));
#16380=CARTESIAN_POINT('Ctrl Pts',(-17.8990654189357,-5.80714485919301,
-12.236639786787));
#16381=CARTESIAN_POINT('Ctrl Pts',(-18.1133511332214,-3.4442934046707,-10.3523286299233));
#16382=CARTESIAN_POINT('Ctrl Pts',(-18.3276368475072,-1.08144195014838,
-8.46801747305968));
#16383=CARTESIAN_POINT('Ctrl Pts',(-18.5419225617929,0.229841679453252,
-5.74510895921686));
#16384=CARTESIAN_POINT('Ctrl Pts',(-18.7562082760786,1.5411253090549,-3.02220044537404));
#16385=CARTESIAN_POINT('Ctrl Pts',(-18.9704939903643,1.5411253090549,-3.46944695195361E-15));
#16386=CARTESIAN_POINT('Ctrl Pts',(-19.18477970465,1.5411253090549,3.02220044537403));
#16387=CARTESIAN_POINT('Ctrl Pts',(-19.3990654189357,0.229841679453252,
5.74510895921686));
#16388=CARTESIAN_POINT('Ctrl Pts',(-19.6133511332214,-1.08144195014837,
8.4680174730597));
#16389=CARTESIAN_POINT('Ctrl Pts',(-19.8276368475071,-3.4442934046707,10.3523286299233));
#16390=CARTESIAN_POINT('Ctrl Pts',(-20.0419225617929,-5.80714485919302,
12.236639786787));
#16391=CARTESIAN_POINT('Ctrl Pts',(-20.2562082760786,-8.75357242959651,
12.9091426524948));
#16392=CARTESIAN_POINT('Ctrl Pts',(-20.4704939903643,-11.7,13.5816455182026));
#16393=CARTESIAN_POINT('Ctrl Pts',(-20.68477970465,-14.6464275704035,12.9091426524948));
#16394=CARTESIAN_POINT('Ctrl Pts',(-20.8990654189357,-17.5928551408069,
12.236639786787));
#16395=CARTESIAN_POINT('Ctrl Pts',(-21.1133511332214,-19.9557065953293,
10.3523286299233));
#16396=CARTESIAN_POINT('Ctrl Pts',(-21.3276368475072,-22.3185580498516,
8.4680174730597));
#16397=CARTESIAN_POINT('Ctrl Pts',(-21.5419225617929,-23.6298416794532,
5.74510895921686));
#16398=CARTESIAN_POINT('Ctrl Pts',(-21.7562082760786,-24.9411253090549,
3.02220044537405));
#16399=CARTESIAN_POINT('Ctrl Pts',(-21.9704939903643,-24.9411253090549,
3.46944695195361E-15));
#16400=CARTESIAN_POINT('Ctrl Pts',(-22.18477970465,-24.9411253090549,-3.02220044537404));
#16401=CARTESIAN_POINT('Ctrl Pts',(-22.3990654189357,-23.6298416794532,
-5.74510895921686));
#16402=CARTESIAN_POINT('Ctrl Pts',(-22.6133511332214,-22.3185580498516,
-8.4680174730597));
#16403=CARTESIAN_POINT('Ctrl Pts',(-22.8276368475072,-19.9557065953293,
-10.3523286299233));
#16404=CARTESIAN_POINT('Ctrl Pts',(-23.0419225617929,-17.592855140807,-12.236639786787));
#16405=CARTESIAN_POINT('Ctrl Pts',(-23.2562082760786,-14.6464275704035,
-12.9091426524948));
#16406=CARTESIAN_POINT('Ctrl Pts',(-23.4704939903643,-11.7,-13.5816455182026));
#16407=CARTESIAN_POINT('Ctrl Pts',(-23.68477970465,-8.75357242959651,-12.9091426524948));
#16408=CARTESIAN_POINT('Ctrl Pts',(-23.8990654189357,-5.80714485919301,
-12.236639786787));
#16409=CARTESIAN_POINT('Ctrl Pts',(-24.1133511332214,-3.4442934046707,-10.3523286299233));
#16410=CARTESIAN_POINT('Ctrl Pts',(-24.3276368475071,-1.08144195014838,
-8.46801747305971));
#16411=CARTESIAN_POINT('Ctrl Pts',(-24.5419225617929,0.229841679453259,
-5.74510895921687));
#16412=CARTESIAN_POINT('Ctrl Pts',(-24.7562082760786,1.54112530905491,-3.02220044537405));
#16413=CARTESIAN_POINT('Ctrl Pts',(-24.9704939903643,1.5411253090549,0.));
#16414=CARTESIAN_POINT('Ctrl Pts',(0.970493990364278,1.5411253090549,-1.38777878078145E-14));
#16415=CARTESIAN_POINT('Ctrl Pts',(0.75620827607856,1.5411253090549,3.02220044537401));
#16416=CARTESIAN_POINT('Ctrl Pts',(0.541922561792848,0.229841679453252,
5.74510895921686));
#16417=CARTESIAN_POINT('Ctrl Pts',(0.327636847507131,-1.08144195014837,
8.4680174730597));
#16418=CARTESIAN_POINT('Ctrl Pts',(0.113351133221419,-3.4442934046707,10.3523286299233));
#16419=CARTESIAN_POINT('Ctrl Pts',(-0.100934581064293,-5.80714485919301,
12.236639786787));
#16420=CARTESIAN_POINT('Ctrl Pts',(-0.315220295350009,-8.7535724295965,
12.9091426524948));
#16421=CARTESIAN_POINT('Ctrl Pts',(-0.529506009635726,-11.7,13.5816455182026));
#16422=CARTESIAN_POINT('Ctrl Pts',(-0.743791723921436,-14.6464275704035,
12.9091426524948));
#16423=CARTESIAN_POINT('Ctrl Pts',(-0.958077438207154,-17.592855140807,
12.236639786787));
#16424=CARTESIAN_POINT('Ctrl Pts',(-1.17236315249287,-19.9557065953293,
10.3523286299233));
#16425=CARTESIAN_POINT('Ctrl Pts',(-1.38664886677858,-22.3185580498516,
8.46801747305969));
#16426=CARTESIAN_POINT('Ctrl Pts',(-1.60093458106429,-23.6298416794532,
5.74510895921685));
#16427=CARTESIAN_POINT('Ctrl Pts',(-1.81522029535001,-24.9411253090549,
3.02220044537403));
#16428=CARTESIAN_POINT('Ctrl Pts',(-2.02950600963573,-24.9411253090549,
-6.93889390390723E-15));
#16429=CARTESIAN_POINT('Ctrl Pts',(-2.24379172392144,-24.9411253090549,
-3.02220044537404));
#16430=CARTESIAN_POINT('Ctrl Pts',(-2.45807743820715,-23.6298416794532,
-5.74510895921686));
#16431=CARTESIAN_POINT('Ctrl Pts',(-2.67236315249287,-22.3185580498516,
-8.4680174730597));
#16432=CARTESIAN_POINT('Ctrl Pts',(-2.88664886677858,-19.9557065953293,
-10.3523286299233));
#16433=CARTESIAN_POINT('Ctrl Pts',(-3.1009345810643,-17.592855140807,-12.236639786787));
#16434=CARTESIAN_POINT('Ctrl Pts',(-3.31522029535001,-14.6464275704035,
-12.9091426524948));
#16435=CARTESIAN_POINT('Ctrl Pts',(-3.52950600963573,-11.7,-13.5816455182026));
#16436=CARTESIAN_POINT('Ctrl Pts',(-3.74379172392144,-8.75357242959649,
-12.9091426524948));
#16437=CARTESIAN_POINT('Ctrl Pts',(-3.95807743820716,-5.80714485919301,
-12.236639786787));
#16438=CARTESIAN_POINT('Ctrl Pts',(-4.17236315249286,-3.44429340467069,
-10.3523286299233));
#16439=CARTESIAN_POINT('Ctrl Pts',(-4.38664886677858,-1.08144195014838,
-8.4680174730597));
#16440=CARTESIAN_POINT('Ctrl Pts',(-4.60093458106429,0.229841679453252,
-5.74510895921687));
#16441=CARTESIAN_POINT('Ctrl Pts',(-4.81522029535001,1.5411253090549,-3.02220044537403));
#16442=CARTESIAN_POINT('Ctrl Pts',(-5.02950600963572,1.5411253090549,0.));
#16443=CARTESIAN_POINT('Ctrl Pts',(-5.24379172392144,1.5411253090549,3.02220044537403));
#16444=CARTESIAN_POINT('Ctrl Pts',(-5.45807743820715,0.229841679453252,
5.74510895921686));
#16445=CARTESIAN_POINT('Ctrl Pts',(-5.67236315249287,-1.08144195014838,
8.4680174730597));
#16446=CARTESIAN_POINT('Ctrl Pts',(-5.88664886677858,-3.4442934046707,10.3523286299233));
#16447=CARTESIAN_POINT('Ctrl Pts',(-6.10093458106429,-5.80714485919302,
12.236639786787));
#16448=CARTESIAN_POINT('Ctrl Pts',(-6.31522029535001,-8.75357242959651,
12.9091426524948));
#16449=CARTESIAN_POINT('Ctrl Pts',(-6.52950600963572,-11.7,13.5816455182026));
#16450=CARTESIAN_POINT('Ctrl Pts',(-6.74379172392143,-14.6464275704035,
12.9091426524948));
#16451=CARTESIAN_POINT('Ctrl Pts',(-6.95807743820715,-17.592855140807,12.2366397867869));
#16452=CARTESIAN_POINT('Ctrl Pts',(-7.17236315249286,-19.9557065953293,
10.3523286299233));
#16453=CARTESIAN_POINT('Ctrl Pts',(-7.38664886677858,-22.3185580498516,
8.46801747305969));
#16454=CARTESIAN_POINT('Ctrl Pts',(-7.6009345810643,-23.6298416794532,5.74510895921687));
#16455=CARTESIAN_POINT('Ctrl Pts',(-7.81522029535001,-24.9411253090549,
3.02220044537403));
#16456=CARTESIAN_POINT('Ctrl Pts',(-8.02950600963572,-24.9411253090549,
-1.38777878078145E-14));
#16457=CARTESIAN_POINT('Ctrl Pts',(-8.24379172392144,-24.9411253090549,
-3.02220044537403));
#16458=CARTESIAN_POINT('Ctrl Pts',(-8.45807743820715,-23.6298416794532,
-5.74510895921687));
#16459=CARTESIAN_POINT('Ctrl Pts',(-8.67236315249287,-22.3185580498516,
-8.46801747305971));
#16460=CARTESIAN_POINT('Ctrl Pts',(-8.88664886677859,-19.9557065953293,
-10.3523286299233));
#16461=CARTESIAN_POINT('Ctrl Pts',(-9.10093458106429,-17.592855140807,-12.236639786787));
#16462=CARTESIAN_POINT('Ctrl Pts',(-9.31522029535001,-14.6464275704035,
-12.9091426524948));
#16463=CARTESIAN_POINT('Ctrl Pts',(-9.52950600963572,-11.7,-13.5816455182026));
#16464=CARTESIAN_POINT('Ctrl Pts',(-9.74379172392145,-8.75357242959651,
-12.9091426524948));
#16465=CARTESIAN_POINT('Ctrl Pts',(-9.95807743820715,-5.80714485919301,
-12.236639786787));
#16466=CARTESIAN_POINT('Ctrl Pts',(-10.1723631524929,-3.4442934046707,-10.3523286299233));
#16467=CARTESIAN_POINT('Ctrl Pts',(-10.3866488667786,-1.08144195014838,
-8.4680174730597));
#16468=CARTESIAN_POINT('Ctrl Pts',(-10.6009345810643,0.229841679453252,
-5.74510895921687));
#16469=CARTESIAN_POINT('Ctrl Pts',(-10.81522029535,1.5411253090549,-3.02220044537404));
#16470=CARTESIAN_POINT('Ctrl Pts',(-11.0295060096357,1.5411253090549,3.46944695195361E-15));
#16471=CARTESIAN_POINT('Ctrl Pts',(-11.2437917239214,1.5411253090549,3.02220044537404));
#16472=CARTESIAN_POINT('Ctrl Pts',(-11.4580774382071,0.229841679453252,
5.74510895921686));
#16473=CARTESIAN_POINT('Ctrl Pts',(-11.6723631524929,-1.08144195014838,
8.4680174730597));
#16474=CARTESIAN_POINT('Ctrl Pts',(-11.8866488667786,-3.4442934046707,10.3523286299233));
#16475=CARTESIAN_POINT('Ctrl Pts',(-12.1009345810643,-5.80714485919302,
12.236639786787));
#16476=CARTESIAN_POINT('Ctrl Pts',(-12.31522029535,-8.75357242959651,12.9091426524948));
#16477=CARTESIAN_POINT('Ctrl Pts',(-12.5295060096357,-11.7,13.5816455182026));
#16478=CARTESIAN_POINT('Ctrl Pts',(-12.7437917239214,-14.6464275704035,
12.9091426524948));
#16479=CARTESIAN_POINT('Ctrl Pts',(-12.9580774382071,-17.5928551408069,
12.236639786787));
#16480=CARTESIAN_POINT('Ctrl Pts',(-13.1723631524929,-19.9557065953293,
10.3523286299233));
#16481=CARTESIAN_POINT('Ctrl Pts',(-13.3866488667786,-22.3185580498516,
8.46801747305969));
#16482=CARTESIAN_POINT('Ctrl Pts',(-13.6009345810643,-23.6298416794532,
5.74510895921686));
#16483=CARTESIAN_POINT('Ctrl Pts',(-13.81522029535,-24.9411253090549,3.02220044537403));
#16484=CARTESIAN_POINT('Ctrl Pts',(-14.0295060096357,-24.9411253090549,
-6.93889390390723E-15));
#16485=CARTESIAN_POINT('Ctrl Pts',(-14.2437917239214,-24.9411253090549,
-3.02220044537403));
#16486=CARTESIAN_POINT('Ctrl Pts',(-14.4580774382072,-23.6298416794532,
-5.74510895921687));
#16487=CARTESIAN_POINT('Ctrl Pts',(-14.6723631524929,-22.3185580498516,
-8.4680174730597));
#16488=CARTESIAN_POINT('Ctrl Pts',(-14.8866488667786,-19.9557065953293,
-10.3523286299233));
#16489=CARTESIAN_POINT('Ctrl Pts',(-15.1009345810643,-17.5928551408069,
-12.236639786787));
#16490=CARTESIAN_POINT('Ctrl Pts',(-15.31522029535,-14.6464275704035,-12.9091426524948));
#16491=CARTESIAN_POINT('Ctrl Pts',(-15.5295060096357,-11.7,-13.5816455182026));
#16492=CARTESIAN_POINT('Ctrl Pts',(-15.7437917239214,-8.75357242959651,
-12.9091426524948));
#16493=CARTESIAN_POINT('Ctrl Pts',(-15.9580774382072,-5.80714485919302,
-12.236639786787));
#16494=CARTESIAN_POINT('Ctrl Pts',(-16.1723631524929,-3.4442934046707,-10.3523286299233));
#16495=CARTESIAN_POINT('Ctrl Pts',(-16.3866488667786,-1.08144195014838,
-8.4680174730597));
#16496=CARTESIAN_POINT('Ctrl Pts',(-16.6009345810643,0.229841679453259,
-5.74510895921687));
#16497=CARTESIAN_POINT('Ctrl Pts',(-16.81522029535,1.5411253090549,-3.02220044537405));
#16498=CARTESIAN_POINT('Ctrl Pts',(-17.0295060096357,1.5411253090549,0.));
#16499=CARTESIAN_POINT('Ctrl Pts',(-17.2437917239215,1.5411253090549,3.02220044537402));
#16500=CARTESIAN_POINT('Ctrl Pts',(-17.4580774382072,0.229841679453259,
5.74510895921687));
#16501=CARTESIAN_POINT('Ctrl Pts',(-17.6723631524929,-1.08144195014838,
8.4680174730597));
#16502=CARTESIAN_POINT('Ctrl Pts',(-17.8866488667786,-3.4442934046707,10.3523286299233));
#16503=CARTESIAN_POINT('Ctrl Pts',(-18.1009345810643,-5.80714485919302,
12.236639786787));
#16504=CARTESIAN_POINT('Ctrl Pts',(-18.31522029535,-8.75357242959651,12.9091426524948));
#16505=CARTESIAN_POINT('Ctrl Pts',(-18.5295060096357,-11.7,13.5816455182026));
#16506=CARTESIAN_POINT('Ctrl Pts',(-18.7437917239214,-14.6464275704035,
12.9091426524948));
#16507=CARTESIAN_POINT('Ctrl Pts',(-18.9580774382072,-17.592855140807,12.236639786787));
#16508=CARTESIAN_POINT('Ctrl Pts',(-19.1723631524929,-19.9557065953293,
10.3523286299233));
#16509=CARTESIAN_POINT('Ctrl Pts',(-19.3866488667786,-22.3185580498516,
8.46801747305969));
#16510=CARTESIAN_POINT('Ctrl Pts',(-19.6009345810643,-23.6298416794532,
5.74510895921686));
#16511=CARTESIAN_POINT('Ctrl Pts',(-19.81522029535,-24.9411253090549,3.02220044537404));
#16512=CARTESIAN_POINT('Ctrl Pts',(-20.0295060096357,-24.9411253090549,
-3.46944695195361E-15));
#16513=CARTESIAN_POINT('Ctrl Pts',(-20.2437917239214,-24.9411253090549,
-3.02220044537404));
#16514=CARTESIAN_POINT('Ctrl Pts',(-20.4580774382072,-23.6298416794532,
-5.74510895921686));
#16515=CARTESIAN_POINT('Ctrl Pts',(-20.6723631524929,-22.3185580498516,
-8.4680174730597));
#16516=CARTESIAN_POINT('Ctrl Pts',(-20.8866488667786,-19.9557065953293,
-10.3523286299233));
#16517=CARTESIAN_POINT('Ctrl Pts',(-21.1009345810643,-17.5928551408069,
-12.236639786787));
#16518=CARTESIAN_POINT('Ctrl Pts',(-21.31522029535,-14.6464275704035,-12.9091426524948));
#16519=CARTESIAN_POINT('Ctrl Pts',(-21.5295060096357,-11.7,-13.5816455182026));
#16520=CARTESIAN_POINT('Ctrl Pts',(-21.7437917239214,-8.7535724295965,-12.9091426524948));
#16521=CARTESIAN_POINT('Ctrl Pts',(-21.9580774382072,-5.80714485919302,
-12.236639786787));
#16522=CARTESIAN_POINT('Ctrl Pts',(-22.1723631524929,-3.4442934046707,-10.3523286299234));
#16523=CARTESIAN_POINT('Ctrl Pts',(-22.3866488667786,-1.08144195014838,
-8.4680174730597));
#16524=CARTESIAN_POINT('Ctrl Pts',(-22.6009345810643,0.229841679453252,
-5.74510895921687));
#16525=CARTESIAN_POINT('Ctrl Pts',(-22.81522029535,1.5411253090549,-3.02220044537406));
#16526=CARTESIAN_POINT('Ctrl Pts',(-23.0295060096357,1.5411253090549,0.));
#16527=CARTESIAN_POINT('Ctrl Pts',(0.654743522119005,2.81197461594778,-1.40439689870177E-14));
#16528=CARTESIAN_POINT('Ctrl Pts',(0.440457807833292,2.81197461594777,3.31226350660556));
#16529=CARTESIAN_POINT('Ctrl Pts',(0.226172093547578,1.37483734075912,6.29650980834649));
#16530=CARTESIAN_POINT('Ctrl Pts',(0.0118863792618643,-0.0622999344295592,
9.28075611008742));
#16531=CARTESIAN_POINT('Ctrl Pts',(-0.20239933502385,-2.65193182212373,
11.3459186275248));
#16532=CARTESIAN_POINT('Ctrl Pts',(-0.416685049309565,-5.24156370981795,
13.4110811449623));
#16533=CARTESIAN_POINT('Ctrl Pts',(-0.630970763595279,-8.47078185490895,
14.1481291139616));
#16534=CARTESIAN_POINT('Ctrl Pts',(-0.84525647788099,-11.7,14.8851770829608));
#16535=CARTESIAN_POINT('Ctrl Pts',(-1.05954219216671,-14.929218145091,14.1481291139616));
#16536=CARTESIAN_POINT('Ctrl Pts',(-1.27382790645242,-18.158436290182,13.4110811449623));
#16537=CARTESIAN_POINT('Ctrl Pts',(-1.48811362073814,-20.7480681778762,
11.3459186275248));
#16538=CARTESIAN_POINT('Ctrl Pts',(-1.70239933502385,-23.3377000655704,
9.2807561100874));
#16539=CARTESIAN_POINT('Ctrl Pts',(-1.91668504930957,-24.7748373407591,
6.29650980834649));
#16540=CARTESIAN_POINT('Ctrl Pts',(-2.13097076359528,-26.2119746159477,
3.31226350660556));
#16541=CARTESIAN_POINT('Ctrl Pts',(-2.345256477881,-26.2119746159478,-1.75549612337721E-14));
#16542=CARTESIAN_POINT('Ctrl Pts',(-2.55954219216671,-26.2119746159478,
-3.31226350660559));
#16543=CARTESIAN_POINT('Ctrl Pts',(-2.77382790645242,-24.7748373407591,
-6.29650980834651));
#16544=CARTESIAN_POINT('Ctrl Pts',(-2.98811362073814,-23.3377000655704,
-9.28075611008743));
#16545=CARTESIAN_POINT('Ctrl Pts',(-3.20239933502385,-20.7480681778762,
-11.3459186275249));
#16546=CARTESIAN_POINT('Ctrl Pts',(-3.41668504930957,-18.158436290182,-13.4110811449623));
#16547=CARTESIAN_POINT('Ctrl Pts',(-3.63097076359528,-14.929218145091,-14.1481291139616));
#16548=CARTESIAN_POINT('Ctrl Pts',(-3.845256477881,-11.7,-14.8851770829609));
#16549=CARTESIAN_POINT('Ctrl Pts',(-4.05954219216671,-8.47078185490897,
-14.1481291139616));
#16550=CARTESIAN_POINT('Ctrl Pts',(-4.27382790645242,-5.24156370981795,
-13.4110811449623));
#16551=CARTESIAN_POINT('Ctrl Pts',(-4.48811362073814,-2.65193182212374,
-11.3459186275249));
#16552=CARTESIAN_POINT('Ctrl Pts',(-4.70239933502385,-0.0622999344295592,
-9.28075611008746));
#16553=CARTESIAN_POINT('Ctrl Pts',(-4.91668504930956,1.37483734075911,-6.29650980834651));
#16554=CARTESIAN_POINT('Ctrl Pts',(-5.13097076359528,2.81197461594777,-3.31226350660559));
#16555=CARTESIAN_POINT('Ctrl Pts',(-5.34525647788099,2.81197461594778,-7.02198449350884E-15));
#16556=CARTESIAN_POINT('Ctrl Pts',(-5.55954219216671,2.81197461594777,3.31226350660558));
#16557=CARTESIAN_POINT('Ctrl Pts',(-5.77382790645242,1.37483734075912,6.29650980834649));
#16558=CARTESIAN_POINT('Ctrl Pts',(-5.98811362073814,-0.0622999344295592,
9.28075611008741));
#16559=CARTESIAN_POINT('Ctrl Pts',(-6.20239933502385,-2.65193182212374,
11.3459186275248));
#16560=CARTESIAN_POINT('Ctrl Pts',(-6.41668504930957,-5.24156370981794,
13.4110811449623));
#16561=CARTESIAN_POINT('Ctrl Pts',(-6.63097076359528,-8.47078185490896,
14.1481291139616));
#16562=CARTESIAN_POINT('Ctrl Pts',(-6.84525647788099,-11.7,14.8851770829608));
#16563=CARTESIAN_POINT('Ctrl Pts',(-7.05954219216671,-14.929218145091,14.1481291139616));
#16564=CARTESIAN_POINT('Ctrl Pts',(-7.27382790645243,-18.158436290182,13.4110811449623));
#16565=CARTESIAN_POINT('Ctrl Pts',(-7.48811362073814,-20.7480681778762,
11.3459186275248));
#16566=CARTESIAN_POINT('Ctrl Pts',(-7.70239933502385,-23.3377000655704,
9.28075611008742));
#16567=CARTESIAN_POINT('Ctrl Pts',(-7.91668504930957,-24.7748373407591,
6.2965098083465));
#16568=CARTESIAN_POINT('Ctrl Pts',(-8.13097076359528,-26.2119746159478,
3.31226350660557));
#16569=CARTESIAN_POINT('Ctrl Pts',(-8.345256477881,-26.2119746159478,-1.75549612337721E-14));
#16570=CARTESIAN_POINT('Ctrl Pts',(-8.55954219216671,-26.2119746159478,
-3.3122635066056));
#16571=CARTESIAN_POINT('Ctrl Pts',(-8.77382790645243,-24.7748373407591,
-6.29650980834652));
#16572=CARTESIAN_POINT('Ctrl Pts',(-8.98811362073814,-23.3377000655704,
-9.28075611008744));
#16573=CARTESIAN_POINT('Ctrl Pts',(-9.20239933502386,-20.7480681778762,
-11.3459186275249));
#16574=CARTESIAN_POINT('Ctrl Pts',(-9.41668504930956,-18.158436290182,-13.4110811449623));
#16575=CARTESIAN_POINT('Ctrl Pts',(-9.63097076359528,-14.929218145091,-14.1481291139616));
#16576=CARTESIAN_POINT('Ctrl Pts',(-9.84525647788099,-11.7,-14.8851770829609));
#16577=CARTESIAN_POINT('Ctrl Pts',(-10.0595421921667,-8.47078185490896,
-14.1481291139616));
#16578=CARTESIAN_POINT('Ctrl Pts',(-10.2738279064524,-5.24156370981796,
-13.4110811449623));
#16579=CARTESIAN_POINT('Ctrl Pts',(-10.4881136207381,-2.65193182212374,
-11.3459186275249));
#16580=CARTESIAN_POINT('Ctrl Pts',(-10.7023993350239,-0.0622999344295592,
-9.28075611008745));
#16581=CARTESIAN_POINT('Ctrl Pts',(-10.9166850493096,1.37483734075912,-6.29650980834652));
#16582=CARTESIAN_POINT('Ctrl Pts',(-11.1309707635953,2.81197461594777,-3.31226350660559));
#16583=CARTESIAN_POINT('Ctrl Pts',(-11.345256477881,2.81197461594778,-2.10659534805265E-14));
#16584=CARTESIAN_POINT('Ctrl Pts',(-11.5595421921667,2.81197461594777,3.31226350660557));
#16585=CARTESIAN_POINT('Ctrl Pts',(-11.7738279064524,1.37483734075912,6.2965098083465));
#16586=CARTESIAN_POINT('Ctrl Pts',(-11.9881136207381,-0.0622999344295592,
9.2807561100874));
#16587=CARTESIAN_POINT('Ctrl Pts',(-12.2023993350239,-2.65193182212374,
11.3459186275248));
#16588=CARTESIAN_POINT('Ctrl Pts',(-12.4166850493096,-5.24156370981794,
13.4110811449623));
#16589=CARTESIAN_POINT('Ctrl Pts',(-12.6309707635953,-8.47078185490896,
14.1481291139616));
#16590=CARTESIAN_POINT('Ctrl Pts',(-12.845256477881,-11.7,14.8851770829609));
#16591=CARTESIAN_POINT('Ctrl Pts',(-13.0595421921667,-14.929218145091,14.1481291139616));
#16592=CARTESIAN_POINT('Ctrl Pts',(-13.2738279064524,-18.158436290182,13.4110811449623));
#16593=CARTESIAN_POINT('Ctrl Pts',(-13.4881136207381,-20.7480681778762,
11.3459186275248));
#16594=CARTESIAN_POINT('Ctrl Pts',(-13.7023993350239,-23.3377000655704,
9.28075611008741));
#16595=CARTESIAN_POINT('Ctrl Pts',(-13.9166850493096,-24.7748373407591,
6.2965098083465));
#16596=CARTESIAN_POINT('Ctrl Pts',(-14.1309707635953,-26.2119746159478,
3.31226350660557));
#16597=CARTESIAN_POINT('Ctrl Pts',(-14.345256477881,-26.2119746159478,-7.02198449350884E-15));
#16598=CARTESIAN_POINT('Ctrl Pts',(-14.5595421921667,-26.2119746159478,
-3.31226350660558));
#16599=CARTESIAN_POINT('Ctrl Pts',(-14.7738279064524,-24.7748373407591,
-6.29650980834651));
#16600=CARTESIAN_POINT('Ctrl Pts',(-14.9881136207381,-23.3377000655704,
-9.28075611008744));
#16601=CARTESIAN_POINT('Ctrl Pts',(-15.2023993350239,-20.7480681778762,
-11.3459186275248));
#16602=CARTESIAN_POINT('Ctrl Pts',(-15.4166850493096,-18.158436290182,-13.4110811449623));
#16603=CARTESIAN_POINT('Ctrl Pts',(-15.6309707635953,-14.929218145091,-14.1481291139616));
#16604=CARTESIAN_POINT('Ctrl Pts',(-15.845256477881,-11.7,-14.8851770829609));
#16605=CARTESIAN_POINT('Ctrl Pts',(-16.0595421921667,-8.47078185490896,
-14.1481291139616));
#16606=CARTESIAN_POINT('Ctrl Pts',(-16.2738279064524,-5.24156370981796,
-13.4110811449623));
#16607=CARTESIAN_POINT('Ctrl Pts',(-16.4881136207381,-2.65193182212374,
-11.3459186275249));
#16608=CARTESIAN_POINT('Ctrl Pts',(-16.7023993350239,-0.0622999344295592,
-9.28075611008745));
#16609=CARTESIAN_POINT('Ctrl Pts',(-16.9166850493096,1.37483734075912,-6.29650980834652));
#16610=CARTESIAN_POINT('Ctrl Pts',(-17.1309707635953,2.81197461594777,-3.3122635066056));
#16611=CARTESIAN_POINT('Ctrl Pts',(-17.345256477881,2.81197461594778,-1.75549612337721E-14));
#16612=CARTESIAN_POINT('Ctrl Pts',(-17.5595421921667,2.81197461594777,3.31226350660556));
#16613=CARTESIAN_POINT('Ctrl Pts',(-17.7738279064524,1.37483734075912,6.29650980834649));
#16614=CARTESIAN_POINT('Ctrl Pts',(-17.9881136207381,-0.0622999344295592,
9.28075611008742));
#16615=CARTESIAN_POINT('Ctrl Pts',(-18.2023993350239,-2.65193182212374,
11.3459186275248));
#16616=CARTESIAN_POINT('Ctrl Pts',(-18.4166850493096,-5.24156370981795,
13.4110811449623));
#16617=CARTESIAN_POINT('Ctrl Pts',(-18.6309707635953,-8.47078185490896,
14.1481291139616));
#16618=CARTESIAN_POINT('Ctrl Pts',(-18.845256477881,-11.7,14.8851770829608));
#16619=CARTESIAN_POINT('Ctrl Pts',(-19.0595421921667,-14.929218145091,14.1481291139616));
#16620=CARTESIAN_POINT('Ctrl Pts',(-19.2738279064524,-18.158436290182,13.4110811449623));
#16621=CARTESIAN_POINT('Ctrl Pts',(-19.4881136207381,-20.7480681778762,
11.3459186275248));
#16622=CARTESIAN_POINT('Ctrl Pts',(-19.7023993350239,-23.3377000655704,
9.28075611008741));
#16623=CARTESIAN_POINT('Ctrl Pts',(-19.9166850493096,-24.7748373407591,
6.29650980834649));
#16624=CARTESIAN_POINT('Ctrl Pts',(-20.1309707635953,-26.2119746159478,
3.31226350660556));
#16625=CARTESIAN_POINT('Ctrl Pts',(-20.345256477881,-26.2119746159478,-1.75549612337721E-14));
#16626=CARTESIAN_POINT('Ctrl Pts',(-20.5595421921667,-26.2119746159478,
-3.31226350660559));
#16627=CARTESIAN_POINT('Ctrl Pts',(-20.7738279064524,-24.7748373407591,
-6.29650980834651));
#16628=CARTESIAN_POINT('Ctrl Pts',(-20.9881136207381,-23.3377000655704,
-9.28075611008743));
#16629=CARTESIAN_POINT('Ctrl Pts',(-21.2023993350239,-20.7480681778762,
-11.3459186275249));
#16630=CARTESIAN_POINT('Ctrl Pts',(-21.4166850493096,-18.158436290182,-13.4110811449623));
#16631=CARTESIAN_POINT('Ctrl Pts',(-21.6309707635953,-14.929218145091,-14.1481291139616));
#16632=CARTESIAN_POINT('Ctrl Pts',(-21.845256477881,-11.7,-14.8851770829609));
#16633=CARTESIAN_POINT('Ctrl Pts',(-22.0595421921667,-8.47078185490896,
-14.1481291139616));
#16634=CARTESIAN_POINT('Ctrl Pts',(-22.2738279064524,-5.24156370981795,
-13.4110811449623));
#16635=CARTESIAN_POINT('Ctrl Pts',(-22.4881136207381,-2.65193182212374,
-11.3459186275249));
#16636=CARTESIAN_POINT('Ctrl Pts',(-22.7023993350238,-0.0622999344295592,
-9.28075611008743));
#16637=CARTESIAN_POINT('Ctrl Pts',(-22.9166850493096,1.37483734075912,-6.29650980834652));
#16638=CARTESIAN_POINT('Ctrl Pts',(-23.1309707635953,2.81197461594777,-3.31226350660561));
#16639=CARTESIAN_POINT('Ctrl Pts',(-23.345256477881,2.81197461594778,-1.40439689870177E-14));
#16640=CARTESIAN_POINT('Ctrl Pts',(-0.65474352211901,2.81197461594778,-2.10659534805265E-14));
#16641=CARTESIAN_POINT('Ctrl Pts',(-0.869029236404722,2.81197461594777,
3.31226350660557));
#16642=CARTESIAN_POINT('Ctrl Pts',(-1.08331495069044,1.37483734075912,6.2965098083465));
#16643=CARTESIAN_POINT('Ctrl Pts',(-1.29760066497615,-0.0622999344295592,
9.28075611008742));
#16644=CARTESIAN_POINT('Ctrl Pts',(-1.51188637926187,-2.65193182212374,
11.3459186275248));
#16645=CARTESIAN_POINT('Ctrl Pts',(-1.72617209354758,-5.24156370981795,
13.4110811449623));
#16646=CARTESIAN_POINT('Ctrl Pts',(-1.94045780783329,-8.47078185490896,
14.1481291139616));
#16647=CARTESIAN_POINT('Ctrl Pts',(-2.15474352211901,-11.7,14.8851770829608));
#16648=CARTESIAN_POINT('Ctrl Pts',(-2.36902923640472,-14.929218145091,14.1481291139616));
#16649=CARTESIAN_POINT('Ctrl Pts',(-2.58331495069044,-18.158436290182,13.4110811449623));
#16650=CARTESIAN_POINT('Ctrl Pts',(-2.79760066497615,-20.7480681778762,
11.3459186275249));
#16651=CARTESIAN_POINT('Ctrl Pts',(-3.01188637926187,-23.3377000655704,
9.28075611008742));
#16652=CARTESIAN_POINT('Ctrl Pts',(-3.22617209354758,-24.7748373407591,
6.2965098083465));
#16653=CARTESIAN_POINT('Ctrl Pts',(-3.4404578078333,-26.2119746159477,3.31226350660556));
#16654=CARTESIAN_POINT('Ctrl Pts',(-3.65474352211901,-26.2119746159478,
-1.75549612337721E-14));
#16655=CARTESIAN_POINT('Ctrl Pts',(-3.86902923640472,-26.2119746159477,
-3.3122635066056));
#16656=CARTESIAN_POINT('Ctrl Pts',(-4.08331495069044,-24.7748373407591,
-6.29650980834652));
#16657=CARTESIAN_POINT('Ctrl Pts',(-4.29760066497615,-23.3377000655704,
-9.28075611008743));
#16658=CARTESIAN_POINT('Ctrl Pts',(-4.51188637926187,-20.7480681778762,
-11.3459186275249));
#16659=CARTESIAN_POINT('Ctrl Pts',(-4.72617209354758,-18.158436290182,-13.4110811449623));
#16660=CARTESIAN_POINT('Ctrl Pts',(-4.94045780783329,-14.929218145091,-14.1481291139616));
#16661=CARTESIAN_POINT('Ctrl Pts',(-5.15474352211901,-11.7,-14.8851770829609));
#16662=CARTESIAN_POINT('Ctrl Pts',(-5.36902923640472,-8.47078185490896,
-14.1481291139616));
#16663=CARTESIAN_POINT('Ctrl Pts',(-5.58331495069044,-5.24156370981795,
-13.4110811449623));
#16664=CARTESIAN_POINT('Ctrl Pts',(-5.79760066497615,-2.65193182212374,
-11.3459186275249));
#16665=CARTESIAN_POINT('Ctrl Pts',(-6.01188637926186,-0.0622999344295592,
-9.28075611008746));
#16666=CARTESIAN_POINT('Ctrl Pts',(-6.22617209354758,1.37483734075912,-6.29650980834653));
#16667=CARTESIAN_POINT('Ctrl Pts',(-6.44045780783329,2.81197461594777,-3.3122635066056));
#16668=CARTESIAN_POINT('Ctrl Pts',(-6.65474352211901,2.81197461594778,-1.40439689870177E-14));
#16669=CARTESIAN_POINT('Ctrl Pts',(-6.86902923640472,2.81197461594777,3.31226350660556));
#16670=CARTESIAN_POINT('Ctrl Pts',(-7.08331495069044,1.37483734075912,6.29650980834649));
#16671=CARTESIAN_POINT('Ctrl Pts',(-7.29760066497615,-0.0622999344295592,
9.28075611008741));
#16672=CARTESIAN_POINT('Ctrl Pts',(-7.51188637926187,-2.65193182212374,
11.3459186275248));
#16673=CARTESIAN_POINT('Ctrl Pts',(-7.72617209354758,-5.24156370981794,
13.4110811449623));
#16674=CARTESIAN_POINT('Ctrl Pts',(-7.9404578078333,-8.47078185490896,14.1481291139616));
#16675=CARTESIAN_POINT('Ctrl Pts',(-8.15474352211901,-11.7,14.8851770829609));
#16676=CARTESIAN_POINT('Ctrl Pts',(-8.36902923640472,-14.929218145091,14.1481291139616));
#16677=CARTESIAN_POINT('Ctrl Pts',(-8.58331495069044,-18.158436290182,13.4110811449623));
#16678=CARTESIAN_POINT('Ctrl Pts',(-8.79760066497615,-20.7480681778762,
11.3459186275248));
#16679=CARTESIAN_POINT('Ctrl Pts',(-9.01188637926186,-23.3377000655704,
9.28075611008741));
#16680=CARTESIAN_POINT('Ctrl Pts',(-9.22617209354758,-24.7748373407591,
6.2965098083465));
#16681=CARTESIAN_POINT('Ctrl Pts',(-9.44045780783329,-26.2119746159478,
3.31226350660557));
#16682=CARTESIAN_POINT('Ctrl Pts',(-9.65474352211901,-26.2119746159478,
-1.05329767402633E-14));
#16683=CARTESIAN_POINT('Ctrl Pts',(-9.86902923640472,-26.2119746159478,
-3.31226350660559));
#16684=CARTESIAN_POINT('Ctrl Pts',(-10.0833149506904,-24.7748373407591,
-6.29650980834652));
#16685=CARTESIAN_POINT('Ctrl Pts',(-10.2976006649762,-23.3377000655704,
-9.28075611008745));
#16686=CARTESIAN_POINT('Ctrl Pts',(-10.5118863792619,-20.7480681778762,
-11.3459186275249));
#16687=CARTESIAN_POINT('Ctrl Pts',(-10.7261720935476,-18.158436290182,-13.4110811449623));
#16688=CARTESIAN_POINT('Ctrl Pts',(-10.9404578078333,-14.929218145091,-14.1481291139616));
#16689=CARTESIAN_POINT('Ctrl Pts',(-11.154743522119,-11.7,-14.8851770829609));
#16690=CARTESIAN_POINT('Ctrl Pts',(-11.3690292364047,-8.47078185490896,
-14.1481291139616));
#16691=CARTESIAN_POINT('Ctrl Pts',(-11.5833149506904,-5.24156370981795,
-13.4110811449623));
#16692=CARTESIAN_POINT('Ctrl Pts',(-11.7976006649762,-2.65193182212373,
-11.3459186275249));
#16693=CARTESIAN_POINT('Ctrl Pts',(-12.0118863792619,-0.0622999344295592,
-9.28075611008745));
#16694=CARTESIAN_POINT('Ctrl Pts',(-12.2261720935476,1.37483734075911,-6.29650980834651));
#16695=CARTESIAN_POINT('Ctrl Pts',(-12.4404578078333,2.81197461594777,-3.3122635066056));
#16696=CARTESIAN_POINT('Ctrl Pts',(-12.654743522119,2.81197461594778,-2.10659534805265E-14));
#16697=CARTESIAN_POINT('Ctrl Pts',(-12.8690292364047,2.81197461594777,3.31226350660555));
#16698=CARTESIAN_POINT('Ctrl Pts',(-13.0833149506904,1.37483734075912,6.2965098083465));
#16699=CARTESIAN_POINT('Ctrl Pts',(-13.2976006649762,-0.0622999344295736,
9.28075611008741));
#16700=CARTESIAN_POINT('Ctrl Pts',(-13.5118863792619,-2.65193182212374,
11.3459186275248));
#16701=CARTESIAN_POINT('Ctrl Pts',(-13.7261720935476,-5.24156370981795,
13.4110811449623));
#16702=CARTESIAN_POINT('Ctrl Pts',(-13.9404578078333,-8.47078185490895,
14.1481291139616));
#16703=CARTESIAN_POINT('Ctrl Pts',(-14.154743522119,-11.7,14.8851770829609));
#16704=CARTESIAN_POINT('Ctrl Pts',(-14.3690292364047,-14.929218145091,14.1481291139616));
#16705=CARTESIAN_POINT('Ctrl Pts',(-14.5833149506904,-18.158436290182,13.4110811449623));
#16706=CARTESIAN_POINT('Ctrl Pts',(-14.7976006649762,-20.7480681778762,
11.3459186275248));
#16707=CARTESIAN_POINT('Ctrl Pts',(-15.0118863792619,-23.3377000655704,
9.28075611008742));
#16708=CARTESIAN_POINT('Ctrl Pts',(-15.2261720935476,-24.7748373407591,
6.29650980834649));
#16709=CARTESIAN_POINT('Ctrl Pts',(-15.4404578078333,-26.2119746159478,
3.31226350660556));
#16710=CARTESIAN_POINT('Ctrl Pts',(-15.654743522119,-26.2119746159477,-7.02198449350884E-15));
#16711=CARTESIAN_POINT('Ctrl Pts',(-15.8690292364047,-26.2119746159478,
-3.31226350660559));
#16712=CARTESIAN_POINT('Ctrl Pts',(-16.0833149506904,-24.7748373407591,
-6.2965098083465));
#16713=CARTESIAN_POINT('Ctrl Pts',(-16.2976006649761,-23.3377000655704,
-9.28075611008744));
#16714=CARTESIAN_POINT('Ctrl Pts',(-16.5118863792619,-20.7480681778762,
-11.3459186275249));
#16715=CARTESIAN_POINT('Ctrl Pts',(-16.7261720935476,-18.158436290182,-13.4110811449623));
#16716=CARTESIAN_POINT('Ctrl Pts',(-16.9404578078333,-14.929218145091,-14.1481291139616));
#16717=CARTESIAN_POINT('Ctrl Pts',(-17.154743522119,-11.7,-14.8851770829609));
#16718=CARTESIAN_POINT('Ctrl Pts',(-17.3690292364047,-8.47078185490896,
-14.1481291139616));
#16719=CARTESIAN_POINT('Ctrl Pts',(-17.5833149506904,-5.24156370981795,
-13.4110811449623));
#16720=CARTESIAN_POINT('Ctrl Pts',(-17.7976006649762,-2.65193182212373,
-11.3459186275249));
#16721=CARTESIAN_POINT('Ctrl Pts',(-18.0118863792619,-0.0622999344295592,
-9.28075611008744));
#16722=CARTESIAN_POINT('Ctrl Pts',(-18.2261720935476,1.37483734075912,-6.29650980834652));
#16723=CARTESIAN_POINT('Ctrl Pts',(-18.4404578078333,2.81197461594777,-3.31226350660559));
#16724=CARTESIAN_POINT('Ctrl Pts',(-18.654743522119,2.81197461594776,-1.05329767402633E-14));
#16725=CARTESIAN_POINT('Ctrl Pts',(-18.8690292364047,2.81197461594777,3.31226350660557));
#16726=CARTESIAN_POINT('Ctrl Pts',(-19.0833149506904,1.37483734075912,6.29650980834649));
#16727=CARTESIAN_POINT('Ctrl Pts',(-19.2976006649762,-0.0622999344295592,
9.28075611008741));
#16728=CARTESIAN_POINT('Ctrl Pts',(-19.5118863792619,-2.65193182212374,
11.3459186275248));
#16729=CARTESIAN_POINT('Ctrl Pts',(-19.7261720935476,-5.24156370981794,
13.4110811449623));
#16730=CARTESIAN_POINT('Ctrl Pts',(-19.9404578078333,-8.47078185490896,
14.1481291139616));
#16731=CARTESIAN_POINT('Ctrl Pts',(-20.154743522119,-11.7,14.8851770829608));
#16732=CARTESIAN_POINT('Ctrl Pts',(-20.3690292364048,-14.929218145091,14.1481291139616));
#16733=CARTESIAN_POINT('Ctrl Pts',(-20.5833149506904,-18.158436290182,13.4110811449623));
#16734=CARTESIAN_POINT('Ctrl Pts',(-20.7976006649762,-20.7480681778762,
11.3459186275248));
#16735=CARTESIAN_POINT('Ctrl Pts',(-21.0118863792619,-23.3377000655704,
9.28075611008741));
#16736=CARTESIAN_POINT('Ctrl Pts',(-21.2261720935476,-24.7748373407591,
6.2965098083465));
#16737=CARTESIAN_POINT('Ctrl Pts',(-21.4404578078333,-26.2119746159477,
3.31226350660557));
#16738=CARTESIAN_POINT('Ctrl Pts',(-21.654743522119,-26.2119746159478,-1.75549612337721E-14));
#16739=CARTESIAN_POINT('Ctrl Pts',(-21.8690292364047,-26.2119746159478,
-3.31226350660559));
#16740=CARTESIAN_POINT('Ctrl Pts',(-22.0833149506904,-24.7748373407591,
-6.29650980834651));
#16741=CARTESIAN_POINT('Ctrl Pts',(-22.2976006649762,-23.3377000655704,
-9.28075611008745));
#16742=CARTESIAN_POINT('Ctrl Pts',(-22.5118863792619,-20.7480681778762,
-11.3459186275249));
#16743=CARTESIAN_POINT('Ctrl Pts',(-22.7261720935476,-18.158436290182,-13.4110811449623));
#16744=CARTESIAN_POINT('Ctrl Pts',(-22.9404578078333,-14.929218145091,-14.1481291139616));
#16745=CARTESIAN_POINT('Ctrl Pts',(-23.154743522119,-11.7,-14.8851770829609));
#16746=CARTESIAN_POINT('Ctrl Pts',(-23.3690292364047,-8.47078185490896,
-14.1481291139616));
#16747=CARTESIAN_POINT('Ctrl Pts',(-23.5833149506904,-5.24156370981795,
-13.4110811449623));
#16748=CARTESIAN_POINT('Ctrl Pts',(-23.7976006649762,-2.65193182212375,
-11.3459186275249));
#16749=CARTESIAN_POINT('Ctrl Pts',(-24.0118863792619,-0.0622999344295592,
-9.28075611008744));
#16750=CARTESIAN_POINT('Ctrl Pts',(-24.2261720935476,1.37483734075912,-6.29650980834651));
#16751=CARTESIAN_POINT('Ctrl Pts',(-24.4404578078333,2.81197461594777,-3.3122635066056));
#16752=CARTESIAN_POINT('Ctrl Pts',(-24.654743522119,2.81197461594778,-1.40439689870177E-14));
#16753=CARTESIAN_POINT('Ctrl Pts',(-0.97049399036428,1.5411253090549,-6.93889390390723E-15));
#16754=CARTESIAN_POINT('Ctrl Pts',(-1.18477970465,1.5411253090549,3.02220044537404));
#16755=CARTESIAN_POINT('Ctrl Pts',(-1.39906541893571,0.229841679453259,
5.74510895921686));
#16756=CARTESIAN_POINT('Ctrl Pts',(-1.61335113322143,-1.08144195014837,
8.46801747305969));
#16757=CARTESIAN_POINT('Ctrl Pts',(-1.82763684750714,-3.4442934046707,10.3523286299233));
#16758=CARTESIAN_POINT('Ctrl Pts',(-2.04192256179286,-5.80714485919302,
12.236639786787));
#16759=CARTESIAN_POINT('Ctrl Pts',(-2.25620827607857,-8.75357242959651,
12.9091426524948));
#16760=CARTESIAN_POINT('Ctrl Pts',(-2.47049399036428,-11.7,13.5816455182026));
#16761=CARTESIAN_POINT('Ctrl Pts',(-2.68477970464999,-14.6464275704035,
12.9091426524948));
#16762=CARTESIAN_POINT('Ctrl Pts',(-2.89906541893571,-17.592855140807,12.236639786787));
#16763=CARTESIAN_POINT('Ctrl Pts',(-3.11335113322142,-19.9557065953293,
10.3523286299233));
#16764=CARTESIAN_POINT('Ctrl Pts',(-3.32763684750714,-22.3185580498516,
8.46801747305969));
#16765=CARTESIAN_POINT('Ctrl Pts',(-3.54192256179285,-23.6298416794532,
5.74510895921685));
#16766=CARTESIAN_POINT('Ctrl Pts',(-3.75620827607857,-24.9411253090549,
3.02220044537403));
#16767=CARTESIAN_POINT('Ctrl Pts',(-3.97049399036428,-24.9411253090549,
-6.93889390390723E-15));
#16768=CARTESIAN_POINT('Ctrl Pts',(-4.18477970464999,-24.9411253090549,
-3.02220044537404));
#16769=CARTESIAN_POINT('Ctrl Pts',(-4.39906541893571,-23.6298416794532,
-5.74510895921685));
#16770=CARTESIAN_POINT('Ctrl Pts',(-4.61335113322142,-22.3185580498516,
-8.46801747305969));
#16771=CARTESIAN_POINT('Ctrl Pts',(-4.82763684750714,-19.9557065953293,
-10.3523286299233));
#16772=CARTESIAN_POINT('Ctrl Pts',(-5.04192256179286,-17.592855140807,-12.236639786787));
#16773=CARTESIAN_POINT('Ctrl Pts',(-5.25620827607857,-14.6464275704035,
-12.9091426524948));
#16774=CARTESIAN_POINT('Ctrl Pts',(-5.47049399036429,-11.7,-13.5816455182026));
#16775=CARTESIAN_POINT('Ctrl Pts',(-5.68477970464999,-8.75357242959651,
-12.9091426524948));
#16776=CARTESIAN_POINT('Ctrl Pts',(-5.89906541893571,-5.80714485919302,
-12.236639786787));
#16777=CARTESIAN_POINT('Ctrl Pts',(-6.11335113322142,-3.4442934046707,-10.3523286299233));
#16778=CARTESIAN_POINT('Ctrl Pts',(-6.32763684750714,-1.08144195014838,
-8.46801747305971));
#16779=CARTESIAN_POINT('Ctrl Pts',(-6.54192256179285,0.229841679453252,
-5.74510895921688));
#16780=CARTESIAN_POINT('Ctrl Pts',(-6.75620827607857,1.5411253090549,-3.02220044537405));
#16781=CARTESIAN_POINT('Ctrl Pts',(-6.97049399036428,1.54112530905488,-6.93889390390723E-15));
#16782=CARTESIAN_POINT('Ctrl Pts',(-7.18477970465,1.5411253090549,3.02220044537401));
#16783=CARTESIAN_POINT('Ctrl Pts',(-7.39906541893571,0.229841679453252,
5.74510895921687));
#16784=CARTESIAN_POINT('Ctrl Pts',(-7.61335113322142,-1.08144195014837,
8.4680174730597));
#16785=CARTESIAN_POINT('Ctrl Pts',(-7.82763684750714,-3.4442934046707,10.3523286299233));
#16786=CARTESIAN_POINT('Ctrl Pts',(-8.04192256179286,-5.80714485919302,
12.236639786787));
#16787=CARTESIAN_POINT('Ctrl Pts',(-8.25620827607856,-8.75357242959651,
12.9091426524948));
#16788=CARTESIAN_POINT('Ctrl Pts',(-8.47049399036428,-11.7,13.5816455182026));
#16789=CARTESIAN_POINT('Ctrl Pts',(-8.68477970464999,-14.6464275704035,
12.9091426524948));
#16790=CARTESIAN_POINT('Ctrl Pts',(-8.89906541893571,-17.592855140807,12.236639786787));
#16791=CARTESIAN_POINT('Ctrl Pts',(-9.11335113322142,-19.9557065953293,
10.3523286299233));
#16792=CARTESIAN_POINT('Ctrl Pts',(-9.32763684750714,-22.3185580498516,
8.4680174730597));
#16793=CARTESIAN_POINT('Ctrl Pts',(-9.54192256179285,-23.6298416794532,
5.74510895921686));
#16794=CARTESIAN_POINT('Ctrl Pts',(-9.75620827607857,-24.9411253090549,
3.02220044537403));
#16795=CARTESIAN_POINT('Ctrl Pts',(-9.97049399036428,-24.9411253090549,
-6.93889390390723E-15));
#16796=CARTESIAN_POINT('Ctrl Pts',(-10.18477970465,-24.9411253090549,-3.02220044537404));
#16797=CARTESIAN_POINT('Ctrl Pts',(-10.3990654189357,-23.6298416794532,
-5.74510895921686));
#16798=CARTESIAN_POINT('Ctrl Pts',(-10.6133511332214,-22.3185580498516,
-8.46801747305971));
#16799=CARTESIAN_POINT('Ctrl Pts',(-10.8276368475071,-19.9557065953293,
-10.3523286299233));
#16800=CARTESIAN_POINT('Ctrl Pts',(-11.0419225617928,-17.5928551408069,
-12.236639786787));
#16801=CARTESIAN_POINT('Ctrl Pts',(-11.2562082760786,-14.6464275704035,
-12.9091426524948));
#16802=CARTESIAN_POINT('Ctrl Pts',(-11.4704939903643,-11.7,-13.5816455182026));
#16803=CARTESIAN_POINT('Ctrl Pts',(-11.68477970465,-8.75357242959649,-12.9091426524948));
#16804=CARTESIAN_POINT('Ctrl Pts',(-11.8990654189357,-5.80714485919302,
-12.236639786787));
#16805=CARTESIAN_POINT('Ctrl Pts',(-12.1133511332214,-3.44429340467069,
-10.3523286299234));
#16806=CARTESIAN_POINT('Ctrl Pts',(-12.3276368475071,-1.08144195014838,
-8.46801747305969));
#16807=CARTESIAN_POINT('Ctrl Pts',(-12.5419225617929,0.229841679453252,
-5.74510895921687));
#16808=CARTESIAN_POINT('Ctrl Pts',(-12.7562082760786,1.54112530905491,-3.02220044537405));
#16809=CARTESIAN_POINT('Ctrl Pts',(-12.9704939903643,1.5411253090549,0.));
#16810=CARTESIAN_POINT('Ctrl Pts',(-13.18477970465,1.5411253090549,3.02220044537401));
#16811=CARTESIAN_POINT('Ctrl Pts',(-13.3990654189357,0.229841679453252,
5.74510895921686));
#16812=CARTESIAN_POINT('Ctrl Pts',(-13.6133511332214,-1.08144195014837,
8.46801747305969));
#16813=CARTESIAN_POINT('Ctrl Pts',(-13.8276368475071,-3.4442934046707,10.3523286299233));
#16814=CARTESIAN_POINT('Ctrl Pts',(-14.0419225617929,-5.80714485919302,
12.236639786787));
#16815=CARTESIAN_POINT('Ctrl Pts',(-14.2562082760786,-8.75357242959651,
12.9091426524948));
#16816=CARTESIAN_POINT('Ctrl Pts',(-14.4704939903643,-11.7,13.5816455182026));
#16817=CARTESIAN_POINT('Ctrl Pts',(-14.68477970465,-14.6464275704035,12.9091426524948));
#16818=CARTESIAN_POINT('Ctrl Pts',(-14.8990654189357,-17.5928551408069,
12.236639786787));
#16819=CARTESIAN_POINT('Ctrl Pts',(-15.1133511332214,-19.9557065953293,
10.3523286299233));
#16820=CARTESIAN_POINT('Ctrl Pts',(-15.3276368475071,-22.3185580498516,
8.46801747305968));
#16821=CARTESIAN_POINT('Ctrl Pts',(-15.5419225617929,-23.6298416794532,
5.74510895921686));
#16822=CARTESIAN_POINT('Ctrl Pts',(-15.7562082760786,-24.9411253090549,
3.02220044537403));
#16823=CARTESIAN_POINT('Ctrl Pts',(-15.9704939903643,-24.9411253090549,
0.));
#16824=CARTESIAN_POINT('Ctrl Pts',(-16.18477970465,-24.9411253090549,-3.02220044537402));
#16825=CARTESIAN_POINT('Ctrl Pts',(-16.3990654189357,-23.6298416794532,
-5.74510895921687));
#16826=CARTESIAN_POINT('Ctrl Pts',(-16.6133511332214,-22.3185580498516,
-8.4680174730597));
#16827=CARTESIAN_POINT('Ctrl Pts',(-16.8276368475071,-19.9557065953293,
-10.3523286299233));
#16828=CARTESIAN_POINT('Ctrl Pts',(-17.0419225617929,-17.5928551408069,
-12.236639786787));
#16829=CARTESIAN_POINT('Ctrl Pts',(-17.2562082760786,-14.6464275704035,
-12.9091426524948));
#16830=CARTESIAN_POINT('Ctrl Pts',(-17.4704939903643,-11.7,-13.5816455182026));
#16831=CARTESIAN_POINT('Ctrl Pts',(-17.68477970465,-8.75357242959651,-12.9091426524948));
#16832=CARTESIAN_POINT('Ctrl Pts',(-17.8990654189357,-5.80714485919301,
-12.236639786787));
#16833=CARTESIAN_POINT('Ctrl Pts',(-18.1133511332214,-3.4442934046707,-10.3523286299233));
#16834=CARTESIAN_POINT('Ctrl Pts',(-18.3276368475072,-1.08144195014838,
-8.46801747305968));
#16835=CARTESIAN_POINT('Ctrl Pts',(-18.5419225617929,0.229841679453252,
-5.74510895921686));
#16836=CARTESIAN_POINT('Ctrl Pts',(-18.7562082760786,1.5411253090549,-3.02220044537404));
#16837=CARTESIAN_POINT('Ctrl Pts',(-18.9704939903643,1.5411253090549,-3.46944695195361E-15));
#16838=CARTESIAN_POINT('Ctrl Pts',(-19.18477970465,1.5411253090549,3.02220044537403));
#16839=CARTESIAN_POINT('Ctrl Pts',(-19.3990654189357,0.229841679453252,
5.74510895921686));
#16840=CARTESIAN_POINT('Ctrl Pts',(-19.6133511332214,-1.08144195014837,
8.4680174730597));
#16841=CARTESIAN_POINT('Ctrl Pts',(-19.8276368475071,-3.4442934046707,10.3523286299233));
#16842=CARTESIAN_POINT('Ctrl Pts',(-20.0419225617929,-5.80714485919302,
12.236639786787));
#16843=CARTESIAN_POINT('Ctrl Pts',(-20.2562082760786,-8.75357242959651,
12.9091426524948));
#16844=CARTESIAN_POINT('Ctrl Pts',(-20.4704939903643,-11.7,13.5816455182026));
#16845=CARTESIAN_POINT('Ctrl Pts',(-20.68477970465,-14.6464275704035,12.9091426524948));
#16846=CARTESIAN_POINT('Ctrl Pts',(-20.8990654189357,-17.5928551408069,
12.236639786787));
#16847=CARTESIAN_POINT('Ctrl Pts',(-21.1133511332214,-19.9557065953293,
10.3523286299233));
#16848=CARTESIAN_POINT('Ctrl Pts',(-21.3276368475072,-22.3185580498516,
8.4680174730597));
#16849=CARTESIAN_POINT('Ctrl Pts',(-21.5419225617929,-23.6298416794532,
5.74510895921686));
#16850=CARTESIAN_POINT('Ctrl Pts',(-21.7562082760786,-24.9411253090549,
3.02220044537405));
#16851=CARTESIAN_POINT('Ctrl Pts',(-21.9704939903643,-24.9411253090549,
3.46944695195361E-15));
#16852=CARTESIAN_POINT('Ctrl Pts',(-22.18477970465,-24.9411253090549,-3.02220044537404));
#16853=CARTESIAN_POINT('Ctrl Pts',(-22.3990654189357,-23.6298416794532,
-5.74510895921686));
#16854=CARTESIAN_POINT('Ctrl Pts',(-22.6133511332214,-22.3185580498516,
-8.4680174730597));
#16855=CARTESIAN_POINT('Ctrl Pts',(-22.8276368475072,-19.9557065953293,
-10.3523286299233));
#16856=CARTESIAN_POINT('Ctrl Pts',(-23.0419225617929,-17.592855140807,-12.236639786787));
#16857=CARTESIAN_POINT('Ctrl Pts',(-23.2562082760786,-14.6464275704035,
-12.9091426524948));
#16858=CARTESIAN_POINT('Ctrl Pts',(-23.4704939903643,-11.7,-13.5816455182026));
#16859=CARTESIAN_POINT('Ctrl Pts',(-23.68477970465,-8.75357242959651,-12.9091426524948));
#16860=CARTESIAN_POINT('Ctrl Pts',(-23.8990654189357,-5.80714485919301,
-12.236639786787));
#16861=CARTESIAN_POINT('Ctrl Pts',(-24.1133511332214,-3.4442934046707,-10.3523286299233));
#16862=CARTESIAN_POINT('Ctrl Pts',(-24.3276368475071,-1.08144195014838,
-8.46801747305971));
#16863=CARTESIAN_POINT('Ctrl Pts',(-24.5419225617929,0.229841679453259,
-5.74510895921687));
#16864=CARTESIAN_POINT('Ctrl Pts',(-24.7562082760786,1.54112530905491,-3.02220044537405));
#16865=CARTESIAN_POINT('Ctrl Pts',(-24.9704939903643,1.5411253090549,0.));
#16866=CARTESIAN_POINT('Ctrl Pts',(0.970493990364278,1.5411253090549,-1.38777878078145E-14));
#16867=CARTESIAN_POINT('Ctrl Pts',(0.75620827607856,1.5411253090549,3.02220044537401));
#16868=CARTESIAN_POINT('Ctrl Pts',(0.541922561792848,0.229841679453252,
5.74510895921686));
#16869=CARTESIAN_POINT('Ctrl Pts',(0.327636847507131,-1.08144195014837,
8.4680174730597));
#16870=CARTESIAN_POINT('Ctrl Pts',(0.113351133221419,-3.4442934046707,10.3523286299233));
#16871=CARTESIAN_POINT('Ctrl Pts',(-0.100934581064293,-5.80714485919301,
12.236639786787));
#16872=CARTESIAN_POINT('Ctrl Pts',(-0.315220295350009,-8.7535724295965,
12.9091426524948));
#16873=CARTESIAN_POINT('Ctrl Pts',(-0.529506009635726,-11.7,13.5816455182026));
#16874=CARTESIAN_POINT('Ctrl Pts',(-0.743791723921436,-14.6464275704035,
12.9091426524948));
#16875=CARTESIAN_POINT('Ctrl Pts',(-0.958077438207154,-17.592855140807,
12.236639786787));
#16876=CARTESIAN_POINT('Ctrl Pts',(-1.17236315249287,-19.9557065953293,
10.3523286299233));
#16877=CARTESIAN_POINT('Ctrl Pts',(-1.38664886677858,-22.3185580498516,
8.46801747305969));
#16878=CARTESIAN_POINT('Ctrl Pts',(-1.60093458106429,-23.6298416794532,
5.74510895921685));
#16879=CARTESIAN_POINT('Ctrl Pts',(-1.81522029535001,-24.9411253090549,
3.02220044537403));
#16880=CARTESIAN_POINT('Ctrl Pts',(-2.02950600963573,-24.9411253090549,
-6.93889390390723E-15));
#16881=CARTESIAN_POINT('Ctrl Pts',(-2.24379172392144,-24.9411253090549,
-3.02220044537404));
#16882=CARTESIAN_POINT('Ctrl Pts',(-2.45807743820715,-23.6298416794532,
-5.74510895921686));
#16883=CARTESIAN_POINT('Ctrl Pts',(-2.67236315249287,-22.3185580498516,
-8.4680174730597));
#16884=CARTESIAN_POINT('Ctrl Pts',(-2.88664886677858,-19.9557065953293,
-10.3523286299233));
#16885=CARTESIAN_POINT('Ctrl Pts',(-3.1009345810643,-17.592855140807,-12.236639786787));
#16886=CARTESIAN_POINT('Ctrl Pts',(-3.31522029535001,-14.6464275704035,
-12.9091426524948));
#16887=CARTESIAN_POINT('Ctrl Pts',(-3.52950600963573,-11.7,-13.5816455182026));
#16888=CARTESIAN_POINT('Ctrl Pts',(-3.74379172392144,-8.75357242959649,
-12.9091426524948));
#16889=CARTESIAN_POINT('Ctrl Pts',(-3.95807743820716,-5.80714485919301,
-12.236639786787));
#16890=CARTESIAN_POINT('Ctrl Pts',(-4.17236315249286,-3.44429340467069,
-10.3523286299233));
#16891=CARTESIAN_POINT('Ctrl Pts',(-4.38664886677858,-1.08144195014838,
-8.4680174730597));
#16892=CARTESIAN_POINT('Ctrl Pts',(-4.60093458106429,0.229841679453252,
-5.74510895921687));
#16893=CARTESIAN_POINT('Ctrl Pts',(-4.81522029535001,1.5411253090549,-3.02220044537403));
#16894=CARTESIAN_POINT('Ctrl Pts',(-5.02950600963572,1.5411253090549,0.));
#16895=CARTESIAN_POINT('Ctrl Pts',(-5.24379172392144,1.5411253090549,3.02220044537403));
#16896=CARTESIAN_POINT('Ctrl Pts',(-5.45807743820715,0.229841679453252,
5.74510895921686));
#16897=CARTESIAN_POINT('Ctrl Pts',(-5.67236315249287,-1.08144195014838,
8.4680174730597));
#16898=CARTESIAN_POINT('Ctrl Pts',(-5.88664886677858,-3.4442934046707,10.3523286299233));
#16899=CARTESIAN_POINT('Ctrl Pts',(-6.10093458106429,-5.80714485919302,
12.236639786787));
#16900=CARTESIAN_POINT('Ctrl Pts',(-6.31522029535001,-8.75357242959651,
12.9091426524948));
#16901=CARTESIAN_POINT('Ctrl Pts',(-6.52950600963572,-11.7,13.5816455182026));
#16902=CARTESIAN_POINT('Ctrl Pts',(-6.74379172392143,-14.6464275704035,
12.9091426524948));
#16903=CARTESIAN_POINT('Ctrl Pts',(-6.95807743820715,-17.592855140807,12.2366397867869));
#16904=CARTESIAN_POINT('Ctrl Pts',(-7.17236315249286,-19.9557065953293,
10.3523286299233));
#16905=CARTESIAN_POINT('Ctrl Pts',(-7.38664886677858,-22.3185580498516,
8.46801747305969));
#16906=CARTESIAN_POINT('Ctrl Pts',(-7.6009345810643,-23.6298416794532,5.74510895921687));
#16907=CARTESIAN_POINT('Ctrl Pts',(-7.81522029535001,-24.9411253090549,
3.02220044537403));
#16908=CARTESIAN_POINT('Ctrl Pts',(-8.02950600963572,-24.9411253090549,
-1.38777878078145E-14));
#16909=CARTESIAN_POINT('Ctrl Pts',(-8.24379172392144,-24.9411253090549,
-3.02220044537403));
#16910=CARTESIAN_POINT('Ctrl Pts',(-8.45807743820715,-23.6298416794532,
-5.74510895921687));
#16911=CARTESIAN_POINT('Ctrl Pts',(-8.67236315249287,-22.3185580498516,
-8.46801747305971));
#16912=CARTESIAN_POINT('Ctrl Pts',(-8.88664886677859,-19.9557065953293,
-10.3523286299233));
#16913=CARTESIAN_POINT('Ctrl Pts',(-9.10093458106429,-17.592855140807,-12.236639786787));
#16914=CARTESIAN_POINT('Ctrl Pts',(-9.31522029535001,-14.6464275704035,
-12.9091426524948));
#16915=CARTESIAN_POINT('Ctrl Pts',(-9.52950600963572,-11.7,-13.5816455182026));
#16916=CARTESIAN_POINT('Ctrl Pts',(-9.74379172392145,-8.75357242959651,
-12.9091426524948));
#16917=CARTESIAN_POINT('Ctrl Pts',(-9.95807743820715,-5.80714485919301,
-12.236639786787));
#16918=CARTESIAN_POINT('Ctrl Pts',(-10.1723631524929,-3.4442934046707,-10.3523286299233));
#16919=CARTESIAN_POINT('Ctrl Pts',(-10.3866488667786,-1.08144195014838,
-8.4680174730597));
#16920=CARTESIAN_POINT('Ctrl Pts',(-10.6009345810643,0.229841679453252,
-5.74510895921687));
#16921=CARTESIAN_POINT('Ctrl Pts',(-10.81522029535,1.5411253090549,-3.02220044537404));
#16922=CARTESIAN_POINT('Ctrl Pts',(-11.0295060096357,1.5411253090549,3.46944695195361E-15));
#16923=CARTESIAN_POINT('Ctrl Pts',(-11.2437917239215,1.5411253090549,3.02220044537404));
#16924=CARTESIAN_POINT('Ctrl Pts',(-11.4580774382071,0.229841679453252,
5.74510895921686));
#16925=CARTESIAN_POINT('Ctrl Pts',(-11.6723631524929,-1.08144195014838,
8.4680174730597));
#16926=CARTESIAN_POINT('Ctrl Pts',(-11.8866488667786,-3.4442934046707,10.3523286299233));
#16927=CARTESIAN_POINT('Ctrl Pts',(-12.1009345810643,-5.80714485919302,
12.236639786787));
#16928=CARTESIAN_POINT('Ctrl Pts',(-12.31522029535,-8.75357242959651,12.9091426524948));
#16929=CARTESIAN_POINT('Ctrl Pts',(-12.5295060096357,-11.7,13.5816455182026));
#16930=CARTESIAN_POINT('Ctrl Pts',(-12.7437917239214,-14.6464275704035,
12.9091426524948));
#16931=CARTESIAN_POINT('Ctrl Pts',(-12.9580774382072,-17.5928551408069,
12.236639786787));
#16932=CARTESIAN_POINT('Ctrl Pts',(-13.1723631524929,-19.9557065953293,
10.3523286299233));
#16933=CARTESIAN_POINT('Ctrl Pts',(-13.3866488667786,-22.3185580498516,
8.46801747305969));
#16934=CARTESIAN_POINT('Ctrl Pts',(-13.6009345810643,-23.6298416794532,
5.74510895921686));
#16935=CARTESIAN_POINT('Ctrl Pts',(-13.81522029535,-24.9411253090549,3.02220044537403));
#16936=CARTESIAN_POINT('Ctrl Pts',(-14.0295060096357,-24.9411253090549,
-6.93889390390723E-15));
#16937=CARTESIAN_POINT('Ctrl Pts',(-14.2437917239214,-24.9411253090549,
-3.02220044537403));
#16938=CARTESIAN_POINT('Ctrl Pts',(-14.4580774382072,-23.6298416794532,
-5.74510895921687));
#16939=CARTESIAN_POINT('Ctrl Pts',(-14.6723631524929,-22.3185580498516,
-8.4680174730597));
#16940=CARTESIAN_POINT('Ctrl Pts',(-14.8866488667786,-19.9557065953293,
-10.3523286299233));
#16941=CARTESIAN_POINT('Ctrl Pts',(-15.1009345810643,-17.5928551408069,
-12.236639786787));
#16942=CARTESIAN_POINT('Ctrl Pts',(-15.31522029535,-14.6464275704035,-12.9091426524948));
#16943=CARTESIAN_POINT('Ctrl Pts',(-15.5295060096357,-11.7,-13.5816455182026));
#16944=CARTESIAN_POINT('Ctrl Pts',(-15.7437917239214,-8.75357242959651,
-12.9091426524948));
#16945=CARTESIAN_POINT('Ctrl Pts',(-15.9580774382072,-5.80714485919302,
-12.236639786787));
#16946=CARTESIAN_POINT('Ctrl Pts',(-16.1723631524929,-3.4442934046707,-10.3523286299233));
#16947=CARTESIAN_POINT('Ctrl Pts',(-16.3866488667786,-1.08144195014838,
-8.4680174730597));
#16948=CARTESIAN_POINT('Ctrl Pts',(-16.6009345810643,0.229841679453259,
-5.74510895921687));
#16949=CARTESIAN_POINT('Ctrl Pts',(-16.81522029535,1.5411253090549,-3.02220044537405));
#16950=CARTESIAN_POINT('Ctrl Pts',(-17.0295060096357,1.5411253090549,0.));
#16951=CARTESIAN_POINT('Ctrl Pts',(-17.2437917239214,1.5411253090549,3.02220044537402));
#16952=CARTESIAN_POINT('Ctrl Pts',(-17.4580774382072,0.229841679453259,
5.74510895921687));
#16953=CARTESIAN_POINT('Ctrl Pts',(-17.6723631524929,-1.08144195014838,
8.4680174730597));
#16954=CARTESIAN_POINT('Ctrl Pts',(-17.8866488667786,-3.4442934046707,10.3523286299233));
#16955=CARTESIAN_POINT('Ctrl Pts',(-18.1009345810643,-5.80714485919302,
12.236639786787));
#16956=CARTESIAN_POINT('Ctrl Pts',(-18.31522029535,-8.75357242959651,12.9091426524948));
#16957=CARTESIAN_POINT('Ctrl Pts',(-18.5295060096357,-11.7,13.5816455182026));
#16958=CARTESIAN_POINT('Ctrl Pts',(-18.7437917239214,-14.6464275704035,
12.9091426524948));
#16959=CARTESIAN_POINT('Ctrl Pts',(-18.9580774382072,-17.592855140807,12.236639786787));
#16960=CARTESIAN_POINT('Ctrl Pts',(-19.1723631524929,-19.9557065953293,
10.3523286299233));
#16961=CARTESIAN_POINT('Ctrl Pts',(-19.3866488667786,-22.3185580498516,
8.46801747305969));
#16962=CARTESIAN_POINT('Ctrl Pts',(-19.6009345810643,-23.6298416794532,
5.74510895921686));
#16963=CARTESIAN_POINT('Ctrl Pts',(-19.81522029535,-24.9411253090549,3.02220044537404));
#16964=CARTESIAN_POINT('Ctrl Pts',(-20.0295060096357,-24.9411253090549,
-3.46944695195361E-15));
#16965=CARTESIAN_POINT('Ctrl Pts',(-20.2437917239214,-24.9411253090549,
-3.02220044537404));
#16966=CARTESIAN_POINT('Ctrl Pts',(-20.4580774382072,-23.6298416794532,
-5.74510895921686));
#16967=CARTESIAN_POINT('Ctrl Pts',(-20.6723631524929,-22.3185580498516,
-8.4680174730597));
#16968=CARTESIAN_POINT('Ctrl Pts',(-20.8866488667786,-19.9557065953293,
-10.3523286299233));
#16969=CARTESIAN_POINT('Ctrl Pts',(-21.1009345810643,-17.5928551408069,
-12.236639786787));
#16970=CARTESIAN_POINT('Ctrl Pts',(-21.31522029535,-14.6464275704035,-12.9091426524948));
#16971=CARTESIAN_POINT('Ctrl Pts',(-21.5295060096357,-11.7,-13.5816455182026));
#16972=CARTESIAN_POINT('Ctrl Pts',(-21.7437917239214,-8.7535724295965,-12.9091426524948));
#16973=CARTESIAN_POINT('Ctrl Pts',(-21.9580774382072,-5.80714485919302,
-12.236639786787));
#16974=CARTESIAN_POINT('Ctrl Pts',(-22.1723631524929,-3.4442934046707,-10.3523286299234));
#16975=CARTESIAN_POINT('Ctrl Pts',(-22.3866488667786,-1.08144195014838,
-8.4680174730597));
#16976=CARTESIAN_POINT('Ctrl Pts',(-22.6009345810643,0.229841679453252,
-5.74510895921687));
#16977=CARTESIAN_POINT('Ctrl Pts',(-22.81522029535,1.5411253090549,-3.02220044537406));
#16978=CARTESIAN_POINT('Ctrl Pts',(-23.0295060096357,1.5411253090549,0.));
#16979=CARTESIAN_POINT('Ctrl Pts',(1.9,-2.19999999999999,0.));
#16980=CARTESIAN_POINT('Ctrl Pts',(1.68571428571428,-2.20000000000001,2.16831300670642));
#16981=CARTESIAN_POINT('Ctrl Pts',(1.47142857142857,-3.14079575492701,4.12189552161678));
#16982=CARTESIAN_POINT('Ctrl Pts',(1.25714285714285,-4.08159150985404,6.07547803652718));
#16983=CARTESIAN_POINT('Ctrl Pts',(1.04285714285714,-5.77684688234202,7.42739908344627));
#16984=CARTESIAN_POINT('Ctrl Pts',(0.828571428571428,-7.47210225483002,
8.77932013036537));
#16985=CARTESIAN_POINT('Ctrl Pts',(0.61428571428571,-9.58605112741501,9.26181516572732));
#16986=CARTESIAN_POINT('Ctrl Pts',(0.399999999999996,-11.7,9.74431020108925));
#16987=CARTESIAN_POINT('Ctrl Pts',(0.185714285714286,-13.813948872585,9.26181516572731));
#16988=CARTESIAN_POINT('Ctrl Pts',(-0.028571428571431,-15.92789774517,8.77932013036537));
#16989=CARTESIAN_POINT('Ctrl Pts',(-0.242857142857143,-17.6231531176579,
7.42739908344628));
#16990=CARTESIAN_POINT('Ctrl Pts',(-0.457142857142861,-19.3184084901459,
6.07547803652717));
#16991=CARTESIAN_POINT('Ctrl Pts',(-0.671428571428574,-20.259204245073,
4.1218955216168));
#16992=CARTESIAN_POINT('Ctrl Pts',(-0.885714285714288,-21.2,2.16831300670641));
#16993=CARTESIAN_POINT('Ctrl Pts',(-1.1,-21.2,0.));
#16994=CARTESIAN_POINT('Ctrl Pts',(-1.31428571428572,-21.2,-2.16831300670643));
#16995=CARTESIAN_POINT('Ctrl Pts',(-1.52857142857143,-20.259204245073,-4.12189552161681));
#16996=CARTESIAN_POINT('Ctrl Pts',(-1.74285714285715,-19.3184084901459,
-6.07547803652718));
#16997=CARTESIAN_POINT('Ctrl Pts',(-1.95714285714286,-17.6231531176579,
-7.42739908344627));
#16998=CARTESIAN_POINT('Ctrl Pts',(-2.17142857142858,-15.92789774517,-8.77932013036537));
#16999=CARTESIAN_POINT('Ctrl Pts',(-2.38571428571429,-13.813948872585,-9.26181516572734));
#17000=CARTESIAN_POINT('Ctrl Pts',(-2.6,-11.7,-9.74431020108928));
#17001=CARTESIAN_POINT('Ctrl Pts',(-2.81428571428572,-9.58605112741501,
-9.26181516572733));
#17002=CARTESIAN_POINT('Ctrl Pts',(-3.02857142857143,-7.47210225483002,
-8.77932013036539));
#17003=CARTESIAN_POINT('Ctrl Pts',(-3.24285714285714,-5.77684688234203,
-7.42739908344628));
#17004=CARTESIAN_POINT('Ctrl Pts',(-3.45714285714286,-4.08159150985404,
-6.07547803652718));
#17005=CARTESIAN_POINT('Ctrl Pts',(-3.67142857142857,-3.14079575492701,
-4.12189552161681));
#17006=CARTESIAN_POINT('Ctrl Pts',(-3.88571428571429,-2.2,-2.16831300670643));
#17007=CARTESIAN_POINT('Ctrl Pts',(-4.1,-2.2,0.));
#17008=CARTESIAN_POINT('Ctrl Pts',(-4.31428571428572,-2.2,2.16831300670642));
#17009=CARTESIAN_POINT('Ctrl Pts',(-4.52857142857143,-3.14079575492702,
4.1218955216168));
#17010=CARTESIAN_POINT('Ctrl Pts',(-4.74285714285714,-4.08159150985404,
6.07547803652717));
#17011=CARTESIAN_POINT('Ctrl Pts',(-4.95714285714286,-5.77684688234202,
7.42739908344626));
#17012=CARTESIAN_POINT('Ctrl Pts',(-5.17142857142857,-7.47210225483002,
8.77932013036537));
#17013=CARTESIAN_POINT('Ctrl Pts',(-5.38571428571428,-9.58605112741501,
9.26181516572731));
#17014=CARTESIAN_POINT('Ctrl Pts',(-5.6,-11.7,9.74431020108925));
#17015=CARTESIAN_POINT('Ctrl Pts',(-5.81428571428572,-13.813948872585,9.26181516572731));
#17016=CARTESIAN_POINT('Ctrl Pts',(-6.02857142857143,-15.9278977451699,
8.77932013036537));
#17017=CARTESIAN_POINT('Ctrl Pts',(-6.24285714285714,-17.623153117658,7.42739908344628));
#17018=CARTESIAN_POINT('Ctrl Pts',(-6.45714285714286,-19.318408490146,6.07547803652718));
#17019=CARTESIAN_POINT('Ctrl Pts',(-6.67142857142857,-20.259204245073,4.12189552161679));
#17020=CARTESIAN_POINT('Ctrl Pts',(-6.88571428571429,-21.2,2.16831300670641));
#17021=CARTESIAN_POINT('Ctrl Pts',(-7.1,-21.2,-1.04083408558608E-14));
#17022=CARTESIAN_POINT('Ctrl Pts',(-7.31428571428571,-21.2,-2.16831300670643));
#17023=CARTESIAN_POINT('Ctrl Pts',(-7.52857142857143,-20.259204245073,-4.1218955216168));
#17024=CARTESIAN_POINT('Ctrl Pts',(-7.74285714285714,-19.3184084901459,
-6.07547803652717));
#17025=CARTESIAN_POINT('Ctrl Pts',(-7.95714285714286,-17.6231531176579,
-7.42739908344627));
#17026=CARTESIAN_POINT('Ctrl Pts',(-8.17142857142857,-15.92789774517,-8.77932013036537));
#17027=CARTESIAN_POINT('Ctrl Pts',(-8.38571428571429,-13.813948872585,-9.26181516572732));
#17028=CARTESIAN_POINT('Ctrl Pts',(-8.6,-11.7,-9.74431020108926));
#17029=CARTESIAN_POINT('Ctrl Pts',(-8.81428571428571,-9.586051127415,-9.26181516572733));
#17030=CARTESIAN_POINT('Ctrl Pts',(-9.02857142857144,-7.47210225483002,
-8.77932013036538));
#17031=CARTESIAN_POINT('Ctrl Pts',(-9.24285714285714,-5.77684688234203,
-7.42739908344628));
#17032=CARTESIAN_POINT('Ctrl Pts',(-9.45714285714286,-4.08159150985404,
-6.07547803652718));
#17033=CARTESIAN_POINT('Ctrl Pts',(-9.67142857142858,-3.14079575492702,
-4.12189552161681));
#17034=CARTESIAN_POINT('Ctrl Pts',(-9.88571428571429,-2.19999999999999,
-2.16831300670644));
#17035=CARTESIAN_POINT('Ctrl Pts',(-10.1,-2.19999999999999,0.));
#17036=CARTESIAN_POINT('Ctrl Pts',(-10.3142857142857,-2.19999999999999,
2.16831300670642));
#17037=CARTESIAN_POINT('Ctrl Pts',(-10.5285714285714,-3.14079575492701,
4.1218955216168));
#17038=CARTESIAN_POINT('Ctrl Pts',(-10.7428571428571,-4.08159150985404,
6.07547803652716));
#17039=CARTESIAN_POINT('Ctrl Pts',(-10.9571428571429,-5.77684688234203,
7.42739908344628));
#17040=CARTESIAN_POINT('Ctrl Pts',(-11.1714285714286,-7.47210225483001,
8.77932013036537));
#17041=CARTESIAN_POINT('Ctrl Pts',(-11.3857142857143,-9.58605112741501,
9.26181516572731));
#17042=CARTESIAN_POINT('Ctrl Pts',(-11.6,-11.7,9.74431020108925));
#17043=CARTESIAN_POINT('Ctrl Pts',(-11.8142857142857,-13.813948872585,9.26181516572731));
#17044=CARTESIAN_POINT('Ctrl Pts',(-12.0285714285714,-15.92789774517,8.77932013036537));
#17045=CARTESIAN_POINT('Ctrl Pts',(-12.2428571428572,-17.6231531176579,
7.42739908344627));
#17046=CARTESIAN_POINT('Ctrl Pts',(-12.4571428571429,-19.3184084901459,
6.07547803652716));
#17047=CARTESIAN_POINT('Ctrl Pts',(-12.6714285714286,-20.259204245073,4.12189552161679));
#17048=CARTESIAN_POINT('Ctrl Pts',(-12.8857142857143,-21.2,2.16831300670642));
#17049=CARTESIAN_POINT('Ctrl Pts',(-13.1,-21.2,-6.93889390390723E-15));
#17050=CARTESIAN_POINT('Ctrl Pts',(-13.3142857142857,-21.2,-2.16831300670643));
#17051=CARTESIAN_POINT('Ctrl Pts',(-13.5285714285714,-20.259204245073,-4.1218955216168));
#17052=CARTESIAN_POINT('Ctrl Pts',(-13.7428571428571,-19.318408490146,-6.07547803652717));
#17053=CARTESIAN_POINT('Ctrl Pts',(-13.9571428571429,-17.623153117658,-7.42739908344627));
#17054=CARTESIAN_POINT('Ctrl Pts',(-14.1714285714286,-15.92789774517,-8.77932013036538));
#17055=CARTESIAN_POINT('Ctrl Pts',(-14.3857142857143,-13.813948872585,-9.26181516572733));
#17056=CARTESIAN_POINT('Ctrl Pts',(-14.6,-11.7,-9.74431020108926));
#17057=CARTESIAN_POINT('Ctrl Pts',(-14.8142857142857,-9.58605112741501,
-9.26181516572732));
#17058=CARTESIAN_POINT('Ctrl Pts',(-15.0285714285714,-7.47210225483002,
-8.77932013036538));
#17059=CARTESIAN_POINT('Ctrl Pts',(-15.2428571428571,-5.77684688234203,
-7.42739908344628));
#17060=CARTESIAN_POINT('Ctrl Pts',(-15.4571428571429,-4.08159150985402,
-6.07547803652717));
#17061=CARTESIAN_POINT('Ctrl Pts',(-15.6714285714286,-3.14079575492701,
-4.12189552161682));
#17062=CARTESIAN_POINT('Ctrl Pts',(-15.8857142857143,-2.19999999999999,
-2.16831300670642));
#17063=CARTESIAN_POINT('Ctrl Pts',(-16.1,-2.20000000000001,-1.38777878078145E-14));
#17064=CARTESIAN_POINT('Ctrl Pts',(-16.3142857142857,-2.19999999999998,
2.16831300670643));
#17065=CARTESIAN_POINT('Ctrl Pts',(-16.5285714285714,-3.14079575492701,
4.12189552161679));
#17066=CARTESIAN_POINT('Ctrl Pts',(-16.7428571428571,-4.08159150985404,
6.07547803652718));
#17067=CARTESIAN_POINT('Ctrl Pts',(-16.9571428571429,-5.77684688234202,
7.42739908344626));
#17068=CARTESIAN_POINT('Ctrl Pts',(-17.1714285714286,-7.47210225483001,
8.77932013036537));
#17069=CARTESIAN_POINT('Ctrl Pts',(-17.3857142857143,-9.58605112741501,
9.26181516572732));
#17070=CARTESIAN_POINT('Ctrl Pts',(-17.6,-11.7,9.74431020108925));
#17071=CARTESIAN_POINT('Ctrl Pts',(-17.8142857142857,-13.813948872585,9.26181516572732));
#17072=CARTESIAN_POINT('Ctrl Pts',(-18.0285714285714,-15.92789774517,8.77932013036538));
#17073=CARTESIAN_POINT('Ctrl Pts',(-18.2428571428571,-17.623153117658,7.42739908344627));
#17074=CARTESIAN_POINT('Ctrl Pts',(-18.4571428571429,-19.318408490146,6.07547803652718));
#17075=CARTESIAN_POINT('Ctrl Pts',(-18.6714285714286,-20.259204245073,4.12189552161679));
#17076=CARTESIAN_POINT('Ctrl Pts',(-18.8857142857143,-21.2,2.16831300670641));
#17077=CARTESIAN_POINT('Ctrl Pts',(-19.1,-21.2,-1.38777878078145E-14));
#17078=CARTESIAN_POINT('Ctrl Pts',(-19.3142857142857,-21.2,-2.16831300670643));
#17079=CARTESIAN_POINT('Ctrl Pts',(-19.5285714285714,-20.259204245073,-4.12189552161681));
#17080=CARTESIAN_POINT('Ctrl Pts',(-19.7428571428572,-19.3184084901459,
-6.07547803652717));
#17081=CARTESIAN_POINT('Ctrl Pts',(-19.9571428571429,-17.623153117658,-7.42739908344628));
#17082=CARTESIAN_POINT('Ctrl Pts',(-20.1714285714286,-15.92789774517,-8.77932013036539));
#17083=CARTESIAN_POINT('Ctrl Pts',(-20.3857142857143,-13.813948872585,-9.26181516572732));
#17084=CARTESIAN_POINT('Ctrl Pts',(-20.6,-11.7,-9.74431020108926));
#17085=CARTESIAN_POINT('Ctrl Pts',(-20.8142857142857,-9.58605112741501,
-9.26181516572732));
#17086=CARTESIAN_POINT('Ctrl Pts',(-21.0285714285714,-7.47210225483001,
-8.77932013036538));
#17087=CARTESIAN_POINT('Ctrl Pts',(-21.2428571428572,-5.77684688234203,
-7.42739908344628));
#17088=CARTESIAN_POINT('Ctrl Pts',(-21.4571428571429,-4.08159150985402,
-6.07547803652718));
#17089=CARTESIAN_POINT('Ctrl Pts',(-21.6714285714286,-3.14079575492701,
-4.1218955216168));
#17090=CARTESIAN_POINT('Ctrl Pts',(-21.8857142857143,-2.20000000000001,
-2.16831300670643));
#17091=CARTESIAN_POINT('Ctrl Pts',(-22.1,-2.20000000000001,-2.08166817117217E-14));
#17092=CARTESIAN_POINT('Ctrl Pts',(0.970493990364278,1.5411253090549,-1.38777878078145E-14));
#17093=CARTESIAN_POINT('Ctrl Pts',(0.75620827607856,1.5411253090549,3.02220044537401));
#17094=CARTESIAN_POINT('Ctrl Pts',(0.541922561792848,0.229841679453252,
5.74510895921686));
#17095=CARTESIAN_POINT('Ctrl Pts',(0.327636847507131,-1.08144195014837,
8.4680174730597));
#17096=CARTESIAN_POINT('Ctrl Pts',(0.113351133221419,-3.4442934046707,10.3523286299233));
#17097=CARTESIAN_POINT('Ctrl Pts',(-0.100934581064293,-5.80714485919301,
12.236639786787));
#17098=CARTESIAN_POINT('Ctrl Pts',(-0.315220295350009,-8.7535724295965,
12.9091426524948));
#17099=CARTESIAN_POINT('Ctrl Pts',(-0.529506009635726,-11.7,13.5816455182026));
#17100=CARTESIAN_POINT('Ctrl Pts',(-0.743791723921436,-14.6464275704035,
12.9091426524948));
#17101=CARTESIAN_POINT('Ctrl Pts',(-0.958077438207154,-17.592855140807,
12.236639786787));
#17102=CARTESIAN_POINT('Ctrl Pts',(-1.17236315249287,-19.9557065953293,
10.3523286299233));
#17103=CARTESIAN_POINT('Ctrl Pts',(-1.38664886677858,-22.3185580498516,
8.46801747305969));
#17104=CARTESIAN_POINT('Ctrl Pts',(-1.60093458106429,-23.6298416794532,
5.74510895921685));
#17105=CARTESIAN_POINT('Ctrl Pts',(-1.81522029535001,-24.9411253090549,
3.02220044537403));
#17106=CARTESIAN_POINT('Ctrl Pts',(-2.02950600963573,-24.9411253090549,
-6.93889390390723E-15));
#17107=CARTESIAN_POINT('Ctrl Pts',(-2.24379172392144,-24.9411253090549,
-3.02220044537404));
#17108=CARTESIAN_POINT('Ctrl Pts',(-2.45807743820715,-23.6298416794532,
-5.74510895921686));
#17109=CARTESIAN_POINT('Ctrl Pts',(-2.67236315249287,-22.3185580498516,
-8.4680174730597));
#17110=CARTESIAN_POINT('Ctrl Pts',(-2.88664886677858,-19.9557065953293,
-10.3523286299233));
#17111=CARTESIAN_POINT('Ctrl Pts',(-3.1009345810643,-17.592855140807,-12.236639786787));
#17112=CARTESIAN_POINT('Ctrl Pts',(-3.31522029535001,-14.6464275704035,
-12.9091426524948));
#17113=CARTESIAN_POINT('Ctrl Pts',(-3.52950600963573,-11.7,-13.5816455182026));
#17114=CARTESIAN_POINT('Ctrl Pts',(-3.74379172392144,-8.75357242959649,
-12.9091426524948));
#17115=CARTESIAN_POINT('Ctrl Pts',(-3.95807743820716,-5.80714485919301,
-12.236639786787));
#17116=CARTESIAN_POINT('Ctrl Pts',(-4.17236315249286,-3.44429340467069,
-10.3523286299233));
#17117=CARTESIAN_POINT('Ctrl Pts',(-4.38664886677858,-1.08144195014838,
-8.4680174730597));
#17118=CARTESIAN_POINT('Ctrl Pts',(-4.60093458106429,0.229841679453252,
-5.74510895921687));
#17119=CARTESIAN_POINT('Ctrl Pts',(-4.81522029535001,1.5411253090549,-3.02220044537403));
#17120=CARTESIAN_POINT('Ctrl Pts',(-5.02950600963572,1.5411253090549,0.));
#17121=CARTESIAN_POINT('Ctrl Pts',(-5.24379172392144,1.5411253090549,3.02220044537403));
#17122=CARTESIAN_POINT('Ctrl Pts',(-5.45807743820715,0.229841679453252,
5.74510895921686));
#17123=CARTESIAN_POINT('Ctrl Pts',(-5.67236315249287,-1.08144195014838,
8.4680174730597));
#17124=CARTESIAN_POINT('Ctrl Pts',(-5.88664886677858,-3.4442934046707,10.3523286299233));
#17125=CARTESIAN_POINT('Ctrl Pts',(-6.10093458106429,-5.80714485919302,
12.236639786787));
#17126=CARTESIAN_POINT('Ctrl Pts',(-6.31522029535001,-8.75357242959651,
12.9091426524948));
#17127=CARTESIAN_POINT('Ctrl Pts',(-6.52950600963572,-11.7,13.5816455182026));
#17128=CARTESIAN_POINT('Ctrl Pts',(-6.74379172392143,-14.6464275704035,
12.9091426524948));
#17129=CARTESIAN_POINT('Ctrl Pts',(-6.95807743820715,-17.592855140807,12.2366397867869));
#17130=CARTESIAN_POINT('Ctrl Pts',(-7.17236315249286,-19.9557065953293,
10.3523286299233));
#17131=CARTESIAN_POINT('Ctrl Pts',(-7.38664886677858,-22.3185580498516,
8.46801747305969));
#17132=CARTESIAN_POINT('Ctrl Pts',(-7.6009345810643,-23.6298416794532,5.74510895921687));
#17133=CARTESIAN_POINT('Ctrl Pts',(-7.81522029535001,-24.9411253090549,
3.02220044537403));
#17134=CARTESIAN_POINT('Ctrl Pts',(-8.02950600963572,-24.9411253090549,
-1.38777878078145E-14));
#17135=CARTESIAN_POINT('Ctrl Pts',(-8.24379172392144,-24.9411253090549,
-3.02220044537403));
#17136=CARTESIAN_POINT('Ctrl Pts',(-8.45807743820715,-23.6298416794532,
-5.74510895921687));
#17137=CARTESIAN_POINT('Ctrl Pts',(-8.67236315249287,-22.3185580498516,
-8.46801747305971));
#17138=CARTESIAN_POINT('Ctrl Pts',(-8.88664886677859,-19.9557065953293,
-10.3523286299233));
#17139=CARTESIAN_POINT('Ctrl Pts',(-9.10093458106429,-17.592855140807,-12.236639786787));
#17140=CARTESIAN_POINT('Ctrl Pts',(-9.31522029535001,-14.6464275704035,
-12.9091426524948));
#17141=CARTESIAN_POINT('Ctrl Pts',(-9.52950600963572,-11.7,-13.5816455182026));
#17142=CARTESIAN_POINT('Ctrl Pts',(-9.74379172392145,-8.75357242959651,
-12.9091426524948));
#17143=CARTESIAN_POINT('Ctrl Pts',(-9.95807743820715,-5.80714485919301,
-12.236639786787));
#17144=CARTESIAN_POINT('Ctrl Pts',(-10.1723631524929,-3.4442934046707,-10.3523286299233));
#17145=CARTESIAN_POINT('Ctrl Pts',(-10.3866488667786,-1.08144195014838,
-8.4680174730597));
#17146=CARTESIAN_POINT('Ctrl Pts',(-10.6009345810643,0.229841679453252,
-5.74510895921687));
#17147=CARTESIAN_POINT('Ctrl Pts',(-10.81522029535,1.5411253090549,-3.02220044537404));
#17148=CARTESIAN_POINT('Ctrl Pts',(-11.0295060096357,1.5411253090549,3.46944695195361E-15));
#17149=CARTESIAN_POINT('Ctrl Pts',(-11.2437917239214,1.5411253090549,3.02220044537404));
#17150=CARTESIAN_POINT('Ctrl Pts',(-11.4580774382071,0.229841679453252,
5.74510895921686));
#17151=CARTESIAN_POINT('Ctrl Pts',(-11.6723631524929,-1.08144195014838,
8.4680174730597));
#17152=CARTESIAN_POINT('Ctrl Pts',(-11.8866488667786,-3.4442934046707,10.3523286299233));
#17153=CARTESIAN_POINT('Ctrl Pts',(-12.1009345810643,-5.80714485919302,
12.236639786787));
#17154=CARTESIAN_POINT('Ctrl Pts',(-12.31522029535,-8.75357242959651,12.9091426524948));
#17155=CARTESIAN_POINT('Ctrl Pts',(-12.5295060096357,-11.7,13.5816455182026));
#17156=CARTESIAN_POINT('Ctrl Pts',(-12.7437917239214,-14.6464275704035,
12.9091426524948));
#17157=CARTESIAN_POINT('Ctrl Pts',(-12.9580774382071,-17.5928551408069,
12.236639786787));
#17158=CARTESIAN_POINT('Ctrl Pts',(-13.1723631524929,-19.9557065953293,
10.3523286299233));
#17159=CARTESIAN_POINT('Ctrl Pts',(-13.3866488667786,-22.3185580498516,
8.46801747305969));
#17160=CARTESIAN_POINT('Ctrl Pts',(-13.6009345810643,-23.6298416794532,
5.74510895921686));
#17161=CARTESIAN_POINT('Ctrl Pts',(-13.81522029535,-24.9411253090549,3.02220044537403));
#17162=CARTESIAN_POINT('Ctrl Pts',(-14.0295060096357,-24.9411253090549,
-6.93889390390723E-15));
#17163=CARTESIAN_POINT('Ctrl Pts',(-14.2437917239214,-24.9411253090549,
-3.02220044537403));
#17164=CARTESIAN_POINT('Ctrl Pts',(-14.4580774382072,-23.6298416794532,
-5.74510895921687));
#17165=CARTESIAN_POINT('Ctrl Pts',(-14.6723631524929,-22.3185580498516,
-8.4680174730597));
#17166=CARTESIAN_POINT('Ctrl Pts',(-14.8866488667786,-19.9557065953293,
-10.3523286299233));
#17167=CARTESIAN_POINT('Ctrl Pts',(-15.1009345810643,-17.5928551408069,
-12.236639786787));
#17168=CARTESIAN_POINT('Ctrl Pts',(-15.31522029535,-14.6464275704035,-12.9091426524948));
#17169=CARTESIAN_POINT('Ctrl Pts',(-15.5295060096357,-11.7,-13.5816455182026));
#17170=CARTESIAN_POINT('Ctrl Pts',(-15.7437917239214,-8.75357242959651,
-12.9091426524948));
#17171=CARTESIAN_POINT('Ctrl Pts',(-15.9580774382072,-5.80714485919302,
-12.236639786787));
#17172=CARTESIAN_POINT('Ctrl Pts',(-16.1723631524929,-3.4442934046707,-10.3523286299233));
#17173=CARTESIAN_POINT('Ctrl Pts',(-16.3866488667786,-1.08144195014838,
-8.4680174730597));
#17174=CARTESIAN_POINT('Ctrl Pts',(-16.6009345810643,0.229841679453259,
-5.74510895921687));
#17175=CARTESIAN_POINT('Ctrl Pts',(-16.81522029535,1.5411253090549,-3.02220044537405));
#17176=CARTESIAN_POINT('Ctrl Pts',(-17.0295060096357,1.5411253090549,0.));
#17177=CARTESIAN_POINT('Ctrl Pts',(-17.2437917239215,1.5411253090549,3.02220044537402));
#17178=CARTESIAN_POINT('Ctrl Pts',(-17.4580774382072,0.229841679453259,
5.74510895921687));
#17179=CARTESIAN_POINT('Ctrl Pts',(-17.6723631524929,-1.08144195014838,
8.4680174730597));
#17180=CARTESIAN_POINT('Ctrl Pts',(-17.8866488667786,-3.4442934046707,10.3523286299233));
#17181=CARTESIAN_POINT('Ctrl Pts',(-18.1009345810643,-5.80714485919302,
12.236639786787));
#17182=CARTESIAN_POINT('Ctrl Pts',(-18.31522029535,-8.75357242959651,12.9091426524948));
#17183=CARTESIAN_POINT('Ctrl Pts',(-18.5295060096357,-11.7,13.5816455182026));
#17184=CARTESIAN_POINT('Ctrl Pts',(-18.7437917239214,-14.6464275704035,
12.9091426524948));
#17185=CARTESIAN_POINT('Ctrl Pts',(-18.9580774382072,-17.592855140807,12.236639786787));
#17186=CARTESIAN_POINT('Ctrl Pts',(-19.1723631524929,-19.9557065953293,
10.3523286299233));
#17187=CARTESIAN_POINT('Ctrl Pts',(-19.3866488667786,-22.3185580498516,
8.46801747305969));
#17188=CARTESIAN_POINT('Ctrl Pts',(-19.6009345810643,-23.6298416794532,
5.74510895921686));
#17189=CARTESIAN_POINT('Ctrl Pts',(-19.81522029535,-24.9411253090549,3.02220044537404));
#17190=CARTESIAN_POINT('Ctrl Pts',(-20.0295060096357,-24.9411253090549,
-3.46944695195361E-15));
#17191=CARTESIAN_POINT('Ctrl Pts',(-20.2437917239214,-24.9411253090549,
-3.02220044537404));
#17192=CARTESIAN_POINT('Ctrl Pts',(-20.4580774382072,-23.6298416794532,
-5.74510895921686));
#17193=CARTESIAN_POINT('Ctrl Pts',(-20.6723631524929,-22.3185580498516,
-8.4680174730597));
#17194=CARTESIAN_POINT('Ctrl Pts',(-20.8866488667786,-19.9557065953293,
-10.3523286299233));
#17195=CARTESIAN_POINT('Ctrl Pts',(-21.1009345810643,-17.5928551408069,
-12.236639786787));
#17196=CARTESIAN_POINT('Ctrl Pts',(-21.31522029535,-14.6464275704035,-12.9091426524948));
#17197=CARTESIAN_POINT('Ctrl Pts',(-21.5295060096357,-11.7,-13.5816455182026));
#17198=CARTESIAN_POINT('Ctrl Pts',(-21.7437917239214,-8.7535724295965,-12.9091426524948));
#17199=CARTESIAN_POINT('Ctrl Pts',(-21.9580774382072,-5.80714485919302,
-12.236639786787));
#17200=CARTESIAN_POINT('Ctrl Pts',(-22.1723631524929,-3.4442934046707,-10.3523286299234));
#17201=CARTESIAN_POINT('Ctrl Pts',(-22.3866488667786,-1.08144195014838,
-8.4680174730597));
#17202=CARTESIAN_POINT('Ctrl Pts',(-22.6009345810643,0.229841679453252,
-5.74510895921687));
#17203=CARTESIAN_POINT('Ctrl Pts',(-22.81522029535,1.5411253090549,-3.02220044537406));
#17204=CARTESIAN_POINT('Ctrl Pts',(-23.0295060096357,1.5411253090549,0.));
#17205=CARTESIAN_POINT('Origin',(128.,-11.7,-3.46944695195361E-15));
#17206=CARTESIAN_POINT('',(128.,-5.19999999999998,-1.62500000000002));
#17207=CARTESIAN_POINT('',(128.,-5.19999999999998,-1.62500000000002));
#17208=CARTESIAN_POINT('',(128.,-5.19999999999998,1.62499999999999));
#17209=CARTESIAN_POINT('',(128.,-5.19999999999998,1.62499999999999));
#17210=CARTESIAN_POINT('',(128.,-5.19999999999998,1.62499999999999));
#17211=CARTESIAN_POINT('Origin',(108.,-5.19999999999998,-1.625));
#17212=CARTESIAN_POINT('',(108.,-5.19999999999998,-1.625));
#17213=CARTESIAN_POINT('',(108.,-5.19999999999998,-1.625));
#17214=CARTESIAN_POINT('',(108.,-5.19999999999998,-1.625));
#17215=CARTESIAN_POINT('Origin',(108.,-5.19999999999998,1.62499999999999));
#17216=CARTESIAN_POINT('',(108.,-5.19999999999998,1.62499999999999));
#17217=CARTESIAN_POINT('',(108.,-5.19999999999998,1.62499999999999));
#17218=CARTESIAN_POINT('',(108.,-5.19999999999998,1.62499999999999));
#17219=CARTESIAN_POINT('Origin',(108.,-5.19999999999998,1.62499999999999));
#17220=CARTESIAN_POINT('',(108.,-5.19999999999998,1.62499999999999));
#17221=CARTESIAN_POINT('Origin',(108.,0.,6.93889390390723E-15));
#17222=CARTESIAN_POINT('Origin',(-58.,-11.7,0.));
#37856=UNCERTAINTY_MEASURE_WITH_UNIT(LENGTH_MEASURE(0.01),#37882,
'DISTANCE_ACCURACY_VALUE',
'Maximum model space distance between geometric entities at asserted c
onnectivities');
#37867=UNCERTAINTY_MEASURE_WITH_UNIT(LENGTH_MEASURE(0.01),#37882,
'DISTANCE_ACCURACY_VALUE',
'Maximum model space distance between geometric entities at asserted c
onnectivities');
#37870=(
GEOMETRIC_REPRESENTATION_CONTEXT(3)
GLOBAL_UNCERTAINTY_ASSIGNED_CONTEXT((#37856))
GLOBAL_UNIT_ASSIGNED_CONTEXT((#37882,#37884,#37885))
REPRESENTATION_CONTEXT('','3D')
);
#37881=(
GEOMETRIC_REPRESENTATION_CONTEXT(3)
GLOBAL_UNCERTAINTY_ASSIGNED_CONTEXT((#37867))
GLOBAL_UNIT_ASSIGNED_CONTEXT((#37882,#37884,#37885))
REPRESENTATION_CONTEXT('','3D')
);
#37882=(
LENGTH_UNIT()
NAMED_UNIT(*)
SI_UNIT(.MILLI.,.METRE.)
);
#37884=(
NAMED_UNIT(*)
PLANE_ANGLE_UNIT()
SI_UNIT($,.RADIAN.)
);
#37885=(
NAMED_UNIT(*)
SI_UNIT($,.STERADIAN.)
SOLID_ANGLE_UNIT()
);
#37888=SHAPE_DEFINITION_REPRESENTATION(#37901,#37955);
#37901=PRODUCT_DEFINITION_SHAPE('',$,#37969);
#37955=SHAPE_REPRESENTATION('',(#11041),#37870);
#37966=PRODUCT_DEFINITION_CONTEXT('part definition',#38007,'design');
#37969=PRODUCT_DEFINITION('PS02','Worm_Shaft',#37982,#37966);
#37982=PRODUCT_DEFINITION_FORMATION('',$,#38011);
#38007=APPLICATION_CONTEXT(
'Core Data for Automotive Mechanical Design Process');
#38008=PRODUCT_CONTEXT('part definition',#38007,'mechanical');
#38011=PRODUCT('PS02','Worm_Shaft',$,(#38008));
#38023=PRESENTATION_STYLE_ASSIGNMENT((#38025));
#38025=SURFACE_STYLE_USAGE(.BOTH.,#38027);
#38027=SURFACE_SIDE_STYLE('',(#38029));
#38029=SURFACE_STYLE_FILL_AREA(#38031);
#38031=FILL_AREA_STYLE('Opaque(202,209,238)',(#38033));
#38033=FILL_AREA_STYLE_COLOUR('Opaque(202,209,238)',#38035);
#38035=COLOUR_RGB('Opaque(202,209,238)', 0.66274510, 0.83137255, 0.94901961);
ENDSEC;
END-ISO-10303-21;
